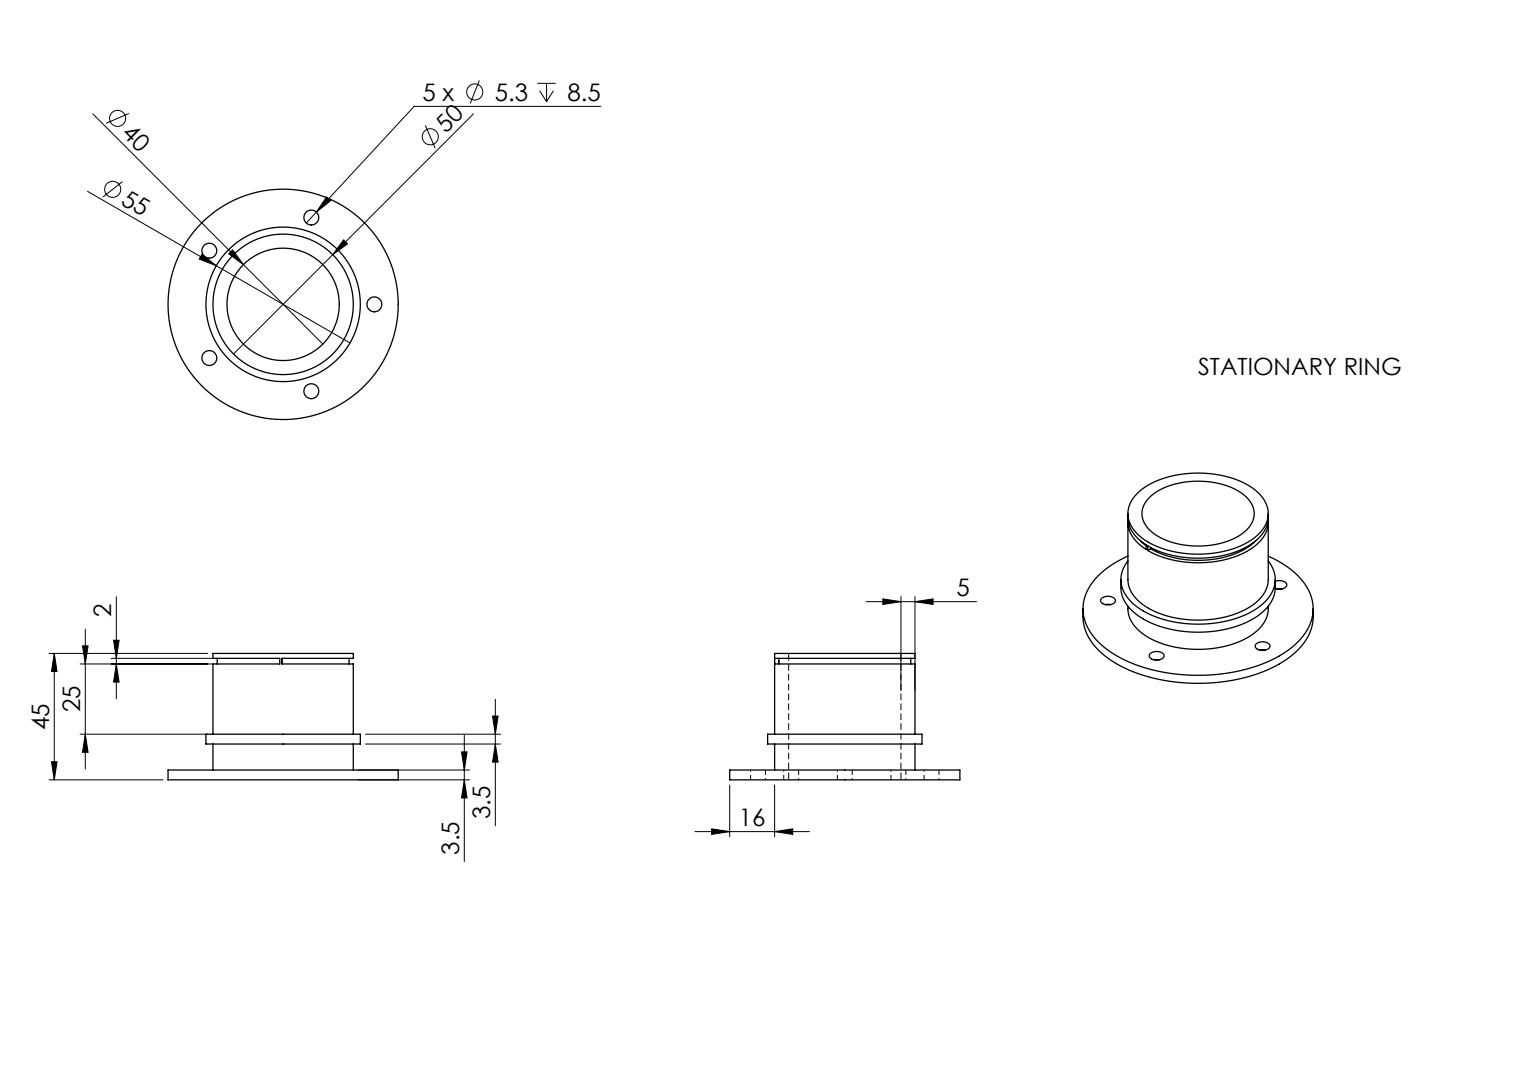
ISO-10303-21;
HEADER;
FILE_DESCRIPTION (('STEP AP214'),
    '1' );
FILE_NAME ('stationary ring.step',
    '2026-10-24T07:08:27',
    ( '' ),
    ( '' ),
    'SwSTEP 2.0',
    'SolidWorks 2026',
    '' );
FILE_SCHEMA (( 'AUTOMOTIVE_DESIGN' ));
ENDSEC;

DATA;
#9=DIRECTION ( 'NONE',  ( 0.000000000000000000, 0.000000000000000000, 1.000000000000000000 ) ) ;
#18=DIRECTION ( 'NONE',  ( 0.000000000000000000, 0.000000000000000000, 1.000000000000000000 ) ) ;
#72=VERTEX_POINT ( 'NONE', #15446 ) ;
#131=ORIENTED_EDGE ( 'NONE', *, *, #5631, .T. ) ;
#137=CARTESIAN_POINT ( 'NONE',  ( -26.29305231718568336, -30.00000000000000000, -19.10302069950552095 ) ) ;
#165=DIRECTION ( 'NONE',  ( 0.000000000000000000, 0.000000000000000000, 1.000000000000000000 ) ) ;
#167=ORIENTED_EDGE ( 'NONE', *, *, #9471, .T. ) ;
#213=CARTESIAN_POINT ( 'NONE',  ( 5.021051876504148963E-15, -26.50000000000000000, 41.00000000000000000 ) ) ;
#243=VERTEX_POINT ( 'NONE', #16663 ) ;
#248=AXIS2_PLACEMENT_3D ( 'NONE', #8151, #16908, #9666 ) ;
#256=EDGE_LOOP ( 'NONE', ( #13526, #15822 ) ) ;
#283=EDGE_CURVE ( 'NONE', #12652, #8705, #12569, .T. ) ;
#288=DIRECTION ( 'NONE',  ( 0.000000000000000000, 0.000000000000000000, 1.000000000000000000 ) ) ;
#294=CIRCLE ( 'NONE', #10631, 2.649999999999999467 ) ;
#295=EDGE_CURVE ( 'NONE', #2351, #16747, #1024, .T. ) ;
#300=CARTESIAN_POINT ( 'NONE',  ( -23.48826165280196321, 13.24999999999999467, -0.7426739052322690604 ) ) ;
#310=EDGE_LOOP ( 'NONE', ( #17511, #1241, #2457, #12125 ) ) ;
#330=ORIENTED_EDGE ( 'NONE', *, *, #18226, .F. ) ;
#331=DIRECTION ( 'NONE',  ( 0.000000000000000000, 0.000000000000000000, 1.000000000000000000 ) ) ;
#333=DIRECTION ( 'NONE',  ( 0.000000000000000000, 1.000000000000000000, 0.000000000000000000 ) ) ;
#368=DIRECTION ( 'NONE',  ( 0.000000000000000000, -0.000000000000000000, -1.000000000000000000 ) ) ;
#403=ORIENTED_EDGE ( 'NONE', *, *, #7543, .T. ) ;
#420=CARTESIAN_POINT ( 'NONE',  ( 32.50000000000000000, -30.00000000000000000, 3.680389326632394941E-13 ) ) ;
#443=DIRECTION ( 'NONE',  ( -0.000000000000000000, 1.000000000000000000, -0.000000000000000000 ) ) ;
#458=DIRECTION ( 'NONE',  ( 0.000000000000000000, 1.000000000000000000, 0.000000000000000000 ) ) ;
#463=CARTESIAN_POINT ( 'NONE',  ( 0.000000000000000000, -30.00000000000000000, 0.000000000000000000 ) ) ;
#468=ORIENTED_EDGE ( 'NONE', *, *, #14255, .T. ) ;
#470=DIRECTION ( 'NONE',  ( 0.000000000000000000, 0.000000000000000000, 1.000000000000000000 ) ) ;
#480=DIRECTION ( 'NONE',  ( 0.000000000000000000, 0.000000000000000000, 1.000000000000000000 ) ) ;
#502=AXIS2_PLACEMENT_3D ( 'NONE', #14003, #960, #12568 ) ;
#505=DIRECTION ( 'NONE',  ( -0.000000000000000000, 1.000000000000000000, -0.000000000000000000 ) ) ;
#522=DIRECTION ( 'NONE',  ( 0.000000000000000000, 0.000000000000000000, 1.000000000000000000 ) ) ;
#528=AXIS2_PLACEMENT_3D ( 'NONE', #15509, #8361, #6654 ) ;
#576=EDGE_LOOP ( 'NONE', ( #11256, #8349, #6691, #4842 ) ) ;
#614=EDGE_LOOP ( 'NONE', ( #7993, #13909, #15314, #4933 ) ) ;
#616=CYLINDRICAL_SURFACE ( 'NONE', #6258, 2.649999999999999467 ) ;
#631=ORIENTED_EDGE ( 'NONE', *, *, #7642, .T. ) ;
#645=VERTEX_POINT ( 'NONE', #15002 ) ;
#647=ADVANCED_FACE ( 'NONE', ( #12940 ), #11765, .T. ) ;
#718=CIRCLE ( 'NONE', #11362, 2.649999999999995914 ) ;
#737=( GEOMETRIC_REPRESENTATION_CONTEXT ( 3 ) GLOBAL_UNCERTAINTY_ASSIGNED_CONTEXT ( ( #6522 ) ) GLOBAL_UNIT_ASSIGNED_CONTEXT ( ( #17644, #7438, #13541 ) ) REPRESENTATION_CONTEXT ( 'NONE', 'WORKASPACE' ) );
#759=ORIENTED_EDGE ( 'NONE', *, *, #6952, .F. ) ;
#769=DIRECTION ( 'NONE',  ( 0.000000000000000000, 0.000000000000000000, 1.000000000000000000 ) ) ;
#786=AXIS2_PLACEMENT_3D ( 'NONE', #10064, #2821, #8624 ) ;
#790=CARTESIAN_POINT ( 'NONE',  ( 32.50000000000000000, -26.50000000000000000, -2.649999999999631317 ) ) ;
#799=DIRECTION ( 'NONE',  ( 1.000000000000000000, 0.000000000000000000, 0.000000000000000000 ) ) ;
#819=CIRCLE ( 'NONE', #9937, 25.00000000000000000 ) ;
#824=EDGE_CURVE ( 'NONE', #3056, #8661, #8769, .T. ) ;
#836=DIRECTION ( 'NONE',  ( 0.9995004958639132076, 0.000000000000000000, 0.03160314490350067673 ) ) ;
#849=DIRECTION ( 'NONE',  ( 0.000000000000000000, 0.000000000000000000, 1.000000000000000000 ) ) ;
#856=FACE_OUTER_BOUND ( 'NONE', #1144, .T. ) ;
#904=DIRECTION ( 'NONE',  ( 0.9995004958639132076, 0.000000000000000000, 0.03160314490350067673 ) ) ;
#911=CARTESIAN_POINT ( 'NONE',  ( 0.000000000000000000, -17.25000000000000355, 0.000000000000000000 ) ) ;
#932=PLANE ( 'NONE',  #17225 ) ;
#960=DIRECTION ( 'NONE',  ( 0.000000000000000000, -1.000000000000000000, 0.000000000000000000 ) ) ;
#995=AXIS2_PLACEMENT_3D ( 'NONE', #17671, #3385, #1944 ) ;
#998=DIRECTION ( 'NONE',  ( 0.000000000000000000, 1.000000000000000000, 0.000000000000000000 ) ) ;
#1008=CARTESIAN_POINT ( 'NONE',  ( 32.50000000000000000, -30.00000000000000000, 3.680389326632394941E-13 ) ) ;
#1009=CIRCLE ( 'NONE', #13174, 2.649999999999999467 ) ;
#1011=CLOSED_SHELL ( 'NONE', ( #7441, #11689, #11568, #2661, #16694, #4242, #6924, #17624, #7600, #3905, #9825, #4801, #9295, #17673, #7168, #6200, #11234, #2883, #16242, #7379, #4112, #1234, #14456, #2013, #11918, #5051, #647, #1767, #1331, #17222, #4597, #7891, #15182 ) ) ;
#1024=CIRCLE ( 'NONE', #4368, 25.00000000000000000 ) ;
#1044=ORIENTED_EDGE ( 'NONE', *, *, #4817, .F. ) ;
#1071=CYLINDRICAL_SURFACE ( 'NONE', #11264, 25.00000000000000000 ) ;
#1090=DIRECTION ( 'NONE',  ( 1.000000000000000000, 0.000000000000000000, 0.000000000000000000 ) ) ;
#1123=DIRECTION ( 'NONE',  ( 0.000000000000000000, 1.000000000000000000, 0.000000000000000000 ) ) ;
#1133=EDGE_LOOP ( 'NONE', ( #14796, #17474, #167, #6880 ) ) ;
#1144=EDGE_LOOP ( 'NONE', ( #12663, #16681, #4780, #9245 ) ) ;
#1149=VECTOR ( 'NONE', #3764, 1000.000000000000000 ) ;
#1163=DIRECTION ( 'NONE',  ( 0.9995004958639132076, 0.000000000000000000, 0.03160314490350067673 ) ) ;
#1178=VERTEX_POINT ( 'NONE', #8655 ) ;
#1208=DIRECTION ( 'NONE',  ( -0.000000000000000000, -1.000000000000000000, 0.000000000000000000 ) ) ;
#1212=CARTESIAN_POINT ( 'NONE',  ( 0.000000000000000000, 15.00000000000000000, 0.000000000000000000 ) ) ;
#1221=ORIENTED_EDGE ( 'NONE', *, *, #283, .T. ) ;
#1233=CIRCLE ( 'NONE', #13693, 2.649999999999999467 ) ;
#1234=ADVANCED_FACE ( 'NONE', ( #6958, #5614 ), #17247, .T. ) ;
#1237=ORIENTED_EDGE ( 'NONE', *, *, #10447, .F. ) ;
#1241=ORIENTED_EDGE ( 'NONE', *, *, #10447, .T. ) ;
#1252=DIRECTION ( 'NONE',  ( -0.000000000000000000, 1.000000000000000000, -0.000000000000000000 ) ) ;
#1253=CARTESIAN_POINT ( 'NONE',  ( 3.061616997868383043E-15, -17.25000000000000355, -25.00000000000000000 ) ) ;
#1268=FACE_OUTER_BOUND ( 'NONE', #15069, .T. ) ;
#1269=CARTESIAN_POINT ( 'NONE',  ( 23.48826165280196321, 13.24999999999999467, 0.7426739052322660628 ) ) ;
#1291=EDGE_CURVE ( 'NONE', #9889, #9794, #9042, .T. ) ;
#1314=ORIENTED_EDGE ( 'NONE', *, *, #6426, .T. ) ;
#1331=ADVANCED_FACE ( 'NONE', ( #10924 ), #16748, .F. ) ;
#1350=COLOUR_RGB ( '',0.8941176470588234615, 0.8941176470588234615, 0.8941176470588234615 ) ;
#1371=VECTOR ( 'NONE', #15439, 1000.000000000000000 ) ;
#1390=CIRCLE ( 'NONE', #4734, 2.649999999999999467 ) ;
#1430=DIRECTION ( 'NONE',  ( 0.000000000000000000, 1.000000000000000000, 0.000000000000000000 ) ) ;
#1433=CARTESIAN_POINT ( 'NONE',  ( 0.000000000000000000, 11.24999999999999645, 0.000000000000000000 ) ) ;
#1466=SHAPE_DEFINITION_REPRESENTATION ( #10584, #16742 ) ;
#1491=VECTOR ( 'NONE', #18744, 1000.000000000000000 ) ;
#1492=CARTESIAN_POINT ( 'NONE',  ( -26.29305231718568336, -30.00000000000000000, -21.75302069950551953 ) ) ;
#1506=ORIENTED_EDGE ( 'NONE', *, *, #17282, .F. ) ;
#1512=ORIENTED_EDGE ( 'NONE', *, *, #4100, .T. ) ;
#1520=CARTESIAN_POINT ( 'NONE',  ( 10.04305231718579705, -26.50000000000000000, 30.90933677959249337 ) ) ;
#1534=VECTOR ( 'NONE', #18328, 1000.000000000000000 ) ;
#1576=EDGE_CURVE ( 'NONE', #16034, #9749, #10261, .T. ) ;
#1646=DIRECTION ( 'NONE',  ( 0.000000000000000000, 1.000000000000000000, 0.000000000000000000 ) ) ;
#1652=FACE_OUTER_BOUND ( 'NONE', #6703, .T. ) ;
#1693=DIRECTION ( 'NONE',  ( 0.000000000000000000, 1.000000000000000000, 0.000000000000000000 ) ) ;
#1729=ORIENTED_EDGE ( 'NONE', *, *, #8148, .T. ) ;
#1735=ORIENTED_EDGE ( 'NONE', *, *, #824, .F. ) ;
#1739=CARTESIAN_POINT ( 'NONE',  ( 10.04305231718605285, -26.50000000000000000, -30.90933677959240811 ) ) ;
#1741=AXIS2_PLACEMENT_3D ( 'NONE', #10000, #3504, #8070 ) ;
#1767=ADVANCED_FACE ( 'NONE', ( #15350 ), #18219, .F. ) ;
#1771=EDGE_CURVE ( 'NONE', #6586, #2692, #8142, .T. ) ;
#1772=CIRCLE ( 'NONE', #8168, 25.00000000000000000 ) ;
#1787=EDGE_CURVE ( 'NONE', #9218, #9749, #16993, .T. ) ;
#1819=FACE_BOUND ( 'NONE', #13502, .T. ) ;
#1822=DIRECTION ( 'NONE',  ( 0.000000000000000000, 0.000000000000000000, 1.000000000000000000 ) ) ;
#1836=LINE ( 'NONE', #14981, #15092 ) ;
#1929=LINE ( 'NONE', #7730, #2930 ) ;
#1944=DIRECTION ( 'NONE',  ( 0.9995004958639130965, 0.000000000000000000, 0.03160314490350068367 ) ) ;
#1955=ORIENTED_EDGE ( 'NONE', *, *, #5164, .T. ) ;
#2013=ADVANCED_FACE ( 'NONE', ( #3443 ), #15158, .T. ) ;
#2032=DIRECTION ( 'NONE',  ( 0.000000000000000000, 0.000000000000000000, 1.000000000000000000 ) ) ;
#2045=DIRECTION ( 'NONE',  ( -0.000000000000000000, 1.000000000000000000, -0.000000000000000000 ) ) ;
#2074=VECTOR ( 'NONE', #10954, 1000.000000000000000 ) ;
#2083=LINE ( 'NONE', #12177, #15046 ) ;
#2131=CARTESIAN_POINT ( 'NONE',  ( 0.000000000000000000, -13.75000000000000355, 27.50000000000000000 ) ) ;
#2161=LINE ( 'NONE', #12448, #9732 ) ;
#2163=CIRCLE ( 'NONE', #10382, 2.649999999999999467 ) ;
#2170=DIRECTION ( 'NONE',  ( 0.000000000000000000, 0.000000000000000000, 1.000000000000000000 ) ) ;
#2173=DIRECTION ( 'NONE',  ( -0.000000000000000000, 1.000000000000000000, -0.000000000000000000 ) ) ;
#2230=CARTESIAN_POINT ( 'NONE',  ( 0.000000000000000000, 15.00000000000000000, 20.00000000000000000 ) ) ;
#2245=CYLINDRICAL_SURFACE ( 'NONE', #9597, 23.50000000000001066 ) ;
#2274=CIRCLE ( 'NONE', #3803, 2.649999999999999467 ) ;
#2277=DIRECTION ( 'NONE',  ( 0.000000000000000000, 0.000000000000000000, 1.000000000000000000 ) ) ;
#2294=VECTOR ( 'NONE', #10245, 1000.000000000000000 ) ;
#2303=DIRECTION ( 'NONE',  ( 0.9995004958639130965, 0.000000000000000000, 0.03160314490350068367 ) ) ;
#2308=CARTESIAN_POINT ( 'NONE',  ( -26.29305231718568336, -30.00000000000000000, -16.45302069950552237 ) ) ;
#2342=ORIENTED_EDGE ( 'NONE', *, *, #6563, .T. ) ;
#2351=VERTEX_POINT ( 'NONE', #1253 ) ;
#2443=CARTESIAN_POINT ( 'NONE',  ( 3.367778697655221307E-15, -13.75000000000000355, -27.50000000000000000 ) ) ;
#2448=DIRECTION ( 'NONE',  ( 0.000000000000000000, 0.000000000000000000, 1.000000000000000000 ) ) ;
#2452=AXIS2_PLACEMENT_3D ( 'NONE', #15849, #11469, #1090 ) ;
#2457=ORIENTED_EDGE ( 'NONE', *, *, #15300, .F. ) ;
#2531=VERTEX_POINT ( 'NONE', #17790 ) ;
#2541=PRODUCT_DEFINITION_CONTEXT ( 'detailed design', #9758, 'design' ) ;
#2549=EDGE_CURVE ( 'NONE', #8661, #3056, #6044, .T. ) ;
#2560=ORIENTED_EDGE ( 'NONE', *, *, #6446, .F. ) ;
#2570=DIRECTION ( 'NONE',  ( -0.000000000000000000, -1.000000000000000000, -0.000000000000000000 ) ) ;
#2582=LINE ( 'NONE', #2690, #16318 ) ;
#2590=EDGE_CURVE ( 'NONE', #5558, #16747, #12648, .T. ) ;
#2595=DIRECTION ( 'NONE',  ( 0.000000000000000000, 0.000000000000000000, 1.000000000000000000 ) ) ;
#2639=ORIENTED_EDGE ( 'NONE', *, *, #16358, .T. ) ;
#2647=ORIENTED_EDGE ( 'NONE', *, *, #6446, .T. ) ;
#2661=ADVANCED_FACE ( 'NONE', ( #856 ), #5123, .F. ) ;
#2677=DIRECTION ( 'NONE',  ( 0.000000000000000000, 0.000000000000000000, 1.000000000000000000 ) ) ;
#2690=CARTESIAN_POINT ( 'NONE',  ( 3.061616997868383043E-15, -30.00000000000000000, -25.00000000000000000 ) ) ;
#2692=VERTEX_POINT ( 'NONE', #11116 ) ;
#2695=DIRECTION ( 'NONE',  ( -0.000000000000000000, 1.000000000000000000, 0.000000000000000000 ) ) ;
#2715=CIRCLE ( 'NONE', #6973, 2.649999999999995914 ) ;
#2720=ORIENTED_EDGE ( 'NONE', *, *, #14352, .F. ) ;
#2723=FACE_OUTER_BOUND ( 'NONE', #12700, .T. ) ;
#2737=DIRECTION ( 'NONE',  ( 0.000000000000000000, 0.000000000000000000, 1.000000000000000000 ) ) ;
#2754=DIRECTION ( 'NONE',  ( 0.000000000000000000, 1.000000000000000000, 0.000000000000000000 ) ) ;
#2764=LINE ( 'NONE', #12948, #2941 ) ;
#2821=DIRECTION ( 'NONE',  ( 0.000000000000000000, -1.000000000000000000, 0.000000000000000000 ) ) ;
#2874=ORIENTED_EDGE ( 'NONE', *, *, #16364, .F. ) ;
#2881=CARTESIAN_POINT ( 'NONE',  ( -26.29305231718568336, -30.00000000000000000, -19.10302069950552095 ) ) ;
#2883=ADVANCED_FACE ( 'NONE', ( #10436 ), #4542, .F. ) ;
#2895=CARTESIAN_POINT ( 'NONE',  ( 2.449293598294706513E-15, 15.00000000000000000, -20.00000000000000000 ) ) ;
#2930=VECTOR ( 'NONE', #505, 1000.000000000000000 ) ;
#2941=VECTOR ( 'NONE', #5714, 1000.000000000000000 ) ;
#3022=CARTESIAN_POINT ( 'NONE',  ( 0.000000000000000000, -13.75000000000000355, 0.000000000000000000 ) ) ;
#3056=VERTEX_POINT ( 'NONE', #13688 ) ;
#3059=CIRCLE ( 'NONE', #10349, 23.50000000000001066 ) ;
#3079=PRESENTATION_STYLE_ASSIGNMENT (( #16125 ) ) ;
#3080=CYLINDRICAL_SURFACE ( 'NONE', #6330, 2.649999999999999467 ) ;
#3083=EDGE_LOOP ( 'NONE', ( #1221, #16532, #13684, #14432, #1506, #13517, #11608, #1237 ) ) ;
#3126=AXIS2_PLACEMENT_3D ( 'NONE', #3946, #13938, #18506 ) ;
#3138=CIRCLE ( 'NONE', #12566, 23.50000000000001066 ) ;
#3162=FILL_AREA_STYLE_COLOUR ( '', #1350 ) ;
#3185=CARTESIAN_POINT ( 'NONE',  ( 0.000000000000000000, -17.25000000000000355, 0.000000000000000000 ) ) ;
#3202=ORIENTED_EDGE ( 'NONE', *, *, #17282, .T. ) ;
#3216=AXIS2_PLACEMENT_3D ( 'NONE', #15972, #12849, #5703 ) ;
#3248=ORIENTED_EDGE ( 'NONE', *, *, #4834, .T. ) ;
#3264=EDGE_CURVE ( 'NONE', #15594, #13366, #11740, .T. ) ;
#3290=ORIENTED_EDGE ( 'NONE', *, *, #16108, .F. ) ;
#3302=EDGE_LOOP ( 'NONE', ( #13752, #17572 ) ) ;
#3347=AXIS2_PLACEMENT_3D ( 'NONE', #5723, #2570, #15537 ) ;
#3363=ORIENTED_EDGE ( 'NONE', *, *, #4070, .F. ) ;
#3385=DIRECTION ( 'NONE',  ( -0.000000000000000000, 1.000000000000000000, 0.000000000000000000 ) ) ;
#3416=DIRECTION ( 'NONE',  ( -0.01515971714484241201, 0.000000000000000000, 0.9998850848853023665 ) ) ;
#3422=FACE_BOUND ( 'NONE', #14128, .T. ) ;
#3429=EDGE_CURVE ( 'NONE', #243, #18412, #12129, .T. ) ;
#3443=FACE_OUTER_BOUND ( 'NONE', #17179, .T. ) ;
#3444=CYLINDRICAL_SURFACE ( 'NONE', #7956, 2.649999999999995914 ) ;
#3449=( NAMED_UNIT ( * ) SI_UNIT ( $, .STERADIAN. ) SOLID_ANGLE_UNIT ( ) );
#3458=( NAMED_UNIT ( * ) SI_UNIT ( $, .STERADIAN. ) SOLID_ANGLE_UNIT ( ) );
#3484=ORIENTED_EDGE ( 'NONE', *, *, #16364, .T. ) ;
#3495=LINE ( 'NONE', #16451, #10796 ) ;
#3503=ORIENTED_EDGE ( 'NONE', *, *, #14588, .T. ) ;
#3504=DIRECTION ( 'NONE',  ( 0.000000000000000000, 1.000000000000000000, 0.000000000000000000 ) ) ;
#3543=AXIS2_PLACEMENT_3D ( 'NONE', #1433, #7237, #18 ) ;
#3561=DIRECTION ( 'NONE',  ( 0.000000000000000000, 0.000000000000000000, 1.000000000000000000 ) ) ;
#3571=CYLINDRICAL_SURFACE ( 'NONE', #5725, 27.50000000000000000 ) ;
#3581=AXIS2_PLACEMENT_3D ( 'NONE', #10797, #9186, #14816 ) ;
#3601=EDGE_CURVE ( 'NONE', #16476, #6965, #11748, .T. ) ;
#3613=VERTEX_POINT ( 'NONE', #16660 ) ;
#3615=DIRECTION ( 'NONE',  ( 0.000000000000000000, 1.000000000000000000, 0.000000000000000000 ) ) ;
#3635=CARTESIAN_POINT ( 'NONE',  ( -26.29305231718584324, -26.50000000000000000, 19.10302069950530779 ) ) ;
#3642=CIRCLE ( 'NONE', #3347, 25.00000000000000000 ) ;
#3660=DIRECTION ( 'NONE',  ( 0.000000000000000000, 1.000000000000000000, 0.000000000000000000 ) ) ;
#3680=UNCERTAINTY_MEASURE_WITH_UNIT (LENGTH_MEASURE( 1.000000000000000082E-05 ), #8870, 'distance_accuracy_value', 'NONE');
#3699=CARTESIAN_POINT ( 'NONE',  ( 32.50000000000000000, -26.50000000000000000, 3.680389326632394941E-13 ) ) ;
#3717=ORIENTED_EDGE ( 'NONE', *, *, #8148, .F. ) ;
#3721=FACE_OUTER_BOUND ( 'NONE', #18727, .T. ) ;
#3764=DIRECTION ( 'NONE',  ( 0.000000000000000000, 1.000000000000000000, 0.000000000000000000 ) ) ;
#3770=ORIENTED_EDGE ( 'NONE', *, *, #2590, .T. ) ;
#3803=AXIS2_PLACEMENT_3D ( 'NONE', #10925, #16749, #2170 ) ;
#3823=AXIS2_PLACEMENT_3D ( 'NONE', #14060, #6530, #11095 ) ;
#3829=DIRECTION ( 'NONE',  ( -0.000000000000000000, -1.000000000000000000, -0.000000000000000000 ) ) ;
#3845=ORIENTED_EDGE ( 'NONE', *, *, #16410, .T. ) ;
#3883=EDGE_CURVE ( 'NONE', #16268, #4068, #5652, .T. ) ;
#3905=ADVANCED_FACE ( 'NONE', ( #17332 ), #13129, .F. ) ;
#3935=CIRCLE ( 'NONE', #13976, 2.649999999999999467 ) ;
#3939=ORIENTED_EDGE ( 'NONE', *, *, #7905, .F. ) ;
#3944=CARTESIAN_POINT ( 'NONE',  ( 32.50000000000000000, -26.50000000000000000, -2.649999999999631317 ) ) ;
#3946=CARTESIAN_POINT ( 'NONE',  ( 0.000000000000000000, -30.00000000000000000, 0.000000000000000000 ) ) ;
#3975=FACE_BOUND ( 'NONE', #256, .T. ) ;
#3998=DIRECTION ( 'NONE',  ( 0.000000000000000000, 0.000000000000000000, 1.000000000000000000 ) ) ;
#4028=EDGE_CURVE ( 'NONE', #13569, #12768, #3495, .T. ) ;
#4044=DIRECTION ( 'NONE',  ( 0.000000000000000000, 0.000000000000000000, 1.000000000000000000 ) ) ;
#4051=ORIENTED_EDGE ( 'NONE', *, *, #18226, .T. ) ;
#4068=VERTEX_POINT ( 'NONE', #6157 ) ;
#4070=EDGE_CURVE ( 'NONE', #4975, #6521, #9290, .T. ) ;
#4100=EDGE_CURVE ( 'NONE', #6721, #12768, #1390, .T. ) ;
#4110=CIRCLE ( 'NONE', #14131, 20.00000000000000000 ) ;
#4112=ADVANCED_FACE ( 'NONE', ( #3975, #9574 ), #932, .F. ) ;
#4125=CARTESIAN_POINT ( 'NONE',  ( 0.000000000000000000, 13.24999999999999467, 0.000000000000000000 ) ) ;
#4131=EDGE_CURVE ( 'NONE', #8705, #8908, #11437, .T. ) ;
#4157=CARTESIAN_POINT ( 'NONE',  ( 0.000000000000000000, -17.25000000000000355, 0.000000000000000000 ) ) ;
#4172=CIRCLE ( 'NONE', #502, 41.00000000000000000 ) ;
#4183=ORIENTED_EDGE ( 'NONE', *, *, #824, .T. ) ;
#4199=DIRECTION ( 'NONE',  ( 0.000000000000000000, 1.000000000000000000, 0.000000000000000000 ) ) ;
#4213=ORIENTED_EDGE ( 'NONE', *, *, #18657, .T. ) ;
#4230=VERTEX_POINT ( 'NONE', #2443 ) ;
#4233=ORIENTED_EDGE ( 'NONE', *, *, #6890, .F. ) ;
#4242=ADVANCED_FACE ( 'NONE', ( #18153 ), #2245, .T. ) ;
#4243=ORIENTED_EDGE ( 'NONE', *, *, #10832, .F. ) ;
#4280=DIRECTION ( 'NONE',  ( 0.000000000000000000, 0.000000000000000000, 1.000000000000000000 ) ) ;
#4308=DIRECTION ( 'NONE',  ( 0.000000000000000000, 0.000000000000000000, -1.000000000000000000 ) ) ;
#4361=DIRECTION ( 'NONE',  ( 0.000000000000000000, 0.000000000000000000, 1.000000000000000000 ) ) ;
#4365=EDGE_CURVE ( 'NONE', #12674, #9439, #5030, .T. ) ;
#4368=AXIS2_PLACEMENT_3D ( 'NONE', #4755, #6278, #10837 ) ;
#4380=DIRECTION ( 'NONE',  ( 0.000000000000000000, -1.000000000000000000, 0.000000000000000000 ) ) ;
#4402=DIRECTION ( 'NONE',  ( 0.000000000000000000, 0.000000000000000000, 1.000000000000000000 ) ) ;
#4404=EDGE_LOOP ( 'NONE', ( #5392, #18272 ) ) ;
#4440=ORIENTED_EDGE ( 'NONE', *, *, #15992, .T. ) ;
#4457=CARTESIAN_POINT ( 'NONE',  ( 0.000000000000000000, 13.24999999999999467, 0.000000000000000000 ) ) ;
#4493=CARTESIAN_POINT ( 'NONE',  ( 0.000000000000000000, -30.00000000000000000, 0.000000000000000000 ) ) ;
#4501=LINE ( 'NONE', #213, #17922 ) ;
#4517=AXIS2_PLACEMENT_3D ( 'NONE', #2881, #10122, #2595 ) ;
#4523=DIRECTION ( 'NONE',  ( 0.000000000000000000, -1.000000000000000000, 0.000000000000000000 ) ) ;
#4542=CYLINDRICAL_SURFACE ( 'NONE', #14192, 20.00000000000000000 ) ;
#4585=FACE_OUTER_BOUND ( 'NONE', #12863, .T. ) ;
#4591=EDGE_CURVE ( 'NONE', #6386, #6721, #12602, .T. ) ;
#4592=DIRECTION ( 'NONE',  ( 0.000000000000000000, 1.000000000000000000, 0.000000000000000000 ) ) ;
#4597=ADVANCED_FACE ( 'NONE', ( #7848 ), #616, .F. ) ;
#4618=ORIENTED_EDGE ( 'NONE', *, *, #13445, .T. ) ;
#4627=ORIENTED_EDGE ( 'NONE', *, *, #2549, .T. ) ;
#4634=ORIENTED_EDGE ( 'NONE', *, *, #6742, .T. ) ;
#4724=CARTESIAN_POINT ( 'NONE',  ( -26.29305231718568336, -26.50000000000000000, -19.10302069950552095 ) ) ;
#4734=AXIS2_PLACEMENT_3D ( 'NONE', #4724, #443, #6356 ) ;
#4755=CARTESIAN_POINT ( 'NONE',  ( 0.000000000000000000, -17.25000000000000355, 0.000000000000000000 ) ) ;
#4775=SURFACE_STYLE_FILL_AREA ( #16406 ) ;
#4776=CARTESIAN_POINT ( 'NONE',  ( 0.000000000000000000, -30.00000000000000000, 25.00000000000000000 ) ) ;
#4780=ORIENTED_EDGE ( 'NONE', *, *, #8755, .T. ) ;
#4785=( LENGTH_UNIT ( ) NAMED_UNIT ( * ) SI_UNIT ( .MILLI., .METRE. ) );
#4793=ORIENTED_EDGE ( 'NONE', *, *, #12813, .F. ) ;
#4797=CARTESIAN_POINT ( 'NONE',  ( 10.04305231718579705, -26.50000000000000000, 30.90933677959249337 ) ) ;
#4801=ADVANCED_FACE ( 'NONE', ( #3721 ), #9518, .T. ) ;
#4817=EDGE_CURVE ( 'NONE', #12768, #6721, #15427, .T. ) ;
#4834=EDGE_CURVE ( 'NONE', #13484, #12910, #4172, .T. ) ;
#4836=DIRECTION ( 'NONE',  ( 0.000000000000000000, 1.000000000000000000, 0.000000000000000000 ) ) ;
#4842=ORIENTED_EDGE ( 'NONE', *, *, #5631, .F. ) ;
#4844=CARTESIAN_POINT ( 'NONE',  ( -26.29305231718584324, -30.00000000000000000, 16.45302069950530566 ) ) ;
#4871=SURFACE_SIDE_STYLE ('',( #4775 ) ) ;
#4893=EDGE_LOOP ( 'NONE', ( #6155, #8486 ) ) ;
#4905=FACE_OUTER_BOUND ( 'NONE', #18171, .T. ) ;
#4918=ORIENTED_EDGE ( 'NONE', *, *, #16108, .T. ) ;
#4933=ORIENTED_EDGE ( 'NONE', *, *, #1576, .T. ) ;
#4957=EDGE_CURVE ( 'NONE', #243, #12652, #2764, .T. ) ;
#4975=VERTEX_POINT ( 'NONE', #10090 ) ;
#5030=CIRCLE ( 'NONE', #16006, 25.00000000000000000 ) ;
#5051=ADVANCED_FACE ( 'NONE', ( #10551 ), #6078, .F. ) ;
#5069=DIRECTION ( 'NONE',  ( -0.000000000000000000, -1.000000000000000000, 0.000000000000000000 ) ) ;
#5077=DIRECTION ( 'NONE',  ( 0.9995004958639132076, 0.000000000000000000, 0.03160314490350067673 ) ) ;
#5123=CYLINDRICAL_SURFACE ( 'NONE', #17011, 2.649999999999995914 ) ;
#5130=ORIENTED_EDGE ( 'NONE', *, *, #4365, .T. ) ;
#5139=DIRECTION ( 'NONE',  ( -0.000000000000000000, 1.000000000000000000, -0.000000000000000000 ) ) ;
#5164=EDGE_CURVE ( 'NONE', #6521, #1178, #17268, .T. ) ;
#5178=ORIENTED_EDGE ( 'NONE', *, *, #4028, .T. ) ;
#5211=CARTESIAN_POINT ( 'NONE',  ( 0.000000000000000000, 15.00000000000000000, 0.000000000000000000 ) ) ;
#5275=AXIS2_PLACEMENT_3D ( 'NONE', #10333, #4523, #7460 ) ;
#5303=LINE ( 'NONE', #11111, #16882 ) ;
#5314=CARTESIAN_POINT ( 'NONE',  ( 10.04305231718605285, -26.50000000000000000, -30.90933677959240811 ) ) ;
#5348=DIRECTION ( 'NONE',  ( 0.000000000000000000, 0.000000000000000000, 1.000000000000000000 ) ) ;
#5356=ADVANCED_BREP_SHAPE_REPRESENTATION ( '', ( #9701, #8017 ), #737 ) ;
#5376=CARTESIAN_POINT ( 'NONE',  ( -26.29305231718584324, -26.50000000000000000, 21.75302069950530637 ) ) ;
#5392=ORIENTED_EDGE ( 'NONE', *, *, #13718, .T. ) ;
#5411=DIRECTION ( 'NONE',  ( 0.9995004958639132076, 0.000000000000000000, 0.03160314490350067673 ) ) ;
#5415=EDGE_LOOP ( 'NONE', ( #13884, #8621, #11743, #1512 ) ) ;
#5428=CARTESIAN_POINT ( 'NONE',  ( 0.000000000000000000, 11.24999999999999645, 0.000000000000000000 ) ) ;
#5435=VERTEX_POINT ( 'NONE', #16374 ) ;
#5447=ORIENTED_EDGE ( 'NONE', *, *, #4957, .F. ) ;
#5456=CIRCLE ( 'NONE', #16092, 25.00000000000000000 ) ;
#5465=CARTESIAN_POINT ( 'NONE',  ( 10.04305231718605285, -30.00000000000000000, -30.90933677959240811 ) ) ;
#5474=DIRECTION ( 'NONE',  ( 0.000000000000000000, 1.000000000000000000, 0.000000000000000000 ) ) ;
#5482=AXIS2_PLACEMENT_3D ( 'NONE', #6517, #15104, #16618 ) ;
#5540=CARTESIAN_POINT ( 'NONE',  ( 0.000000000000000000, 11.24999999999999467, 0.000000000000000000 ) ) ;
#5558=VERTEX_POINT ( 'NONE', #8176 ) ;
#5581=ORIENTED_EDGE ( 'NONE', *, *, #2590, .F. ) ;
#5596=DIRECTION ( 'NONE',  ( 0.000000000000000000, 1.000000000000000000, 0.000000000000000000 ) ) ;
#5614=FACE_OUTER_BOUND ( 'NONE', #8466, .T. ) ;
#5631=EDGE_CURVE ( 'NONE', #17331, #9794, #7105, .T. ) ;
#5632=ORIENTED_EDGE ( 'NONE', *, *, #18805, .T. ) ;
#5637=CIRCLE ( 'NONE', #16281, 2.649999999999995914 ) ;
#5652=CIRCLE ( 'NONE', #3216, 2.649999999999999467 ) ;
#5703=DIRECTION ( 'NONE',  ( 0.000000000000000000, 0.000000000000000000, 1.000000000000000000 ) ) ;
#5714=DIRECTION ( 'NONE',  ( 0.000000000000000000, 1.000000000000000000, 0.000000000000000000 ) ) ;
#5723=CARTESIAN_POINT ( 'NONE',  ( 0.000000000000000000, 11.24999999999999645, 0.000000000000000000 ) ) ;
#5725=AXIS2_PLACEMENT_3D ( 'NONE', #911, #15469, #11065 ) ;
#5756=EDGE_LOOP ( 'NONE', ( #3363, #759, #1729, #4634 ) ) ;
#5810=CARTESIAN_POINT ( 'NONE',  ( 0.000000000000000000, -26.50000000000000000, 0.000000000000000000 ) ) ;
#5830=DIRECTION ( 'NONE',  ( 0.000000000000000000, 0.000000000000000000, 1.000000000000000000 ) ) ;
#5834=DIRECTION ( 'NONE',  ( -0.000000000000000000, -1.000000000000000000, -0.000000000000000000 ) ) ;
#5914=DIRECTION ( 'NONE',  ( 0.000000000000000000, 1.000000000000000000, 0.000000000000000000 ) ) ;
#5926=DIRECTION ( 'NONE',  ( 0.000000000000000000, 1.000000000000000000, 0.000000000000000000 ) ) ;
#5970=CIRCLE ( 'NONE', #8416, 41.00000000000000000 ) ;
#5975=ORIENTED_EDGE ( 'NONE', *, *, #12831, .F. ) ;
#5982=FACE_OUTER_BOUND ( 'NONE', #17091, .T. ) ;
#5985=CYLINDRICAL_SURFACE ( 'NONE', #13306, 2.649999999999999467 ) ;
#5992=EDGE_CURVE ( 'NONE', #17369, #72, #16669, .T. ) ;
#5996=AXIS2_PLACEMENT_3D ( 'NONE', #1520, #15553, #9 ) ;
#6044=CIRCLE ( 'NONE', #13043, 20.00000000000000000 ) ;
#6061=CARTESIAN_POINT ( 'NONE',  ( 0.000000000000000000, -30.00000000000000000, 0.000000000000000000 ) ) ;
#6066=CARTESIAN_POINT ( 'NONE',  ( 10.04305231718579705, -26.50000000000000000, 28.25933677959249835 ) ) ;
#6069=ORIENTED_EDGE ( 'NONE', *, *, #8644, .F. ) ;
#6077=EDGE_LOOP ( 'NONE', ( #10014, #4213 ) ) ;
#6078=PLANE ( 'NONE',  #16629 ) ;
#6109=EDGE_LOOP ( 'NONE', ( #12115, #2874 ) ) ;
#6126=CYLINDRICAL_SURFACE ( 'NONE', #14673, 2.649999999999999467 ) ;
#6152=DIRECTION ( 'NONE',  ( 0.000000000000000000, 1.000000000000000000, 0.000000000000000000 ) ) ;
#6155=ORIENTED_EDGE ( 'NONE', *, *, #14448, .F. ) ;
#6157=CARTESIAN_POINT ( 'NONE',  ( -26.29305231718584324, -30.00000000000000000, 21.75302069950530637 ) ) ;
#6162=AXIS2_PLACEMENT_3D ( 'NONE', #9836, #5069, #904 ) ;
#6179=CARTESIAN_POINT ( 'NONE',  ( -26.29305231718584324, -26.50000000000000000, 19.10302069950530779 ) ) ;
#6183=CARTESIAN_POINT ( 'NONE',  ( 0.000000000000000000, 13.24999999999999822, 0.000000000000000000 ) ) ;
#6200=ADVANCED_FACE ( 'NONE', ( #13563 ), #16423, .T. ) ;
#6201=SHAPE_REPRESENTATION_RELATIONSHIP ( 'NONE' , 'NONE' ,  #16742, #5356 ) ;
#6223=DIRECTION ( 'NONE',  ( 0.000000000000000000, 0.000000000000000000, 1.000000000000000000 ) ) ;
#6258=AXIS2_PLACEMENT_3D ( 'NONE', #6421, #7938, #8029 ) ;
#6264=AXIS2_PLACEMENT_3D ( 'NONE', #10502, #8804, #331 ) ;
#6278=DIRECTION ( 'NONE',  ( -0.000000000000000000, -1.000000000000000000, -0.000000000000000000 ) ) ;
#6298=ORIENTED_EDGE ( 'NONE', *, *, #18060, .T. ) ;
#6307=AXIS2_PLACEMENT_3D ( 'NONE', #4797, #12028, #6223 ) ;
#6309=DIRECTION ( 'NONE',  ( -0.000000000000000000, -1.000000000000000000, -0.000000000000000000 ) ) ;
#6330=AXIS2_PLACEMENT_3D ( 'NONE', #17816, #14883, #10315 ) ;
#6356=DIRECTION ( 'NONE',  ( 0.000000000000000000, 0.000000000000000000, 1.000000000000000000 ) ) ;
#6386=VERTEX_POINT ( 'NONE', #2308 ) ;
#6391=CARTESIAN_POINT ( 'NONE',  ( -1.200950573245989306, 13.24999999999999822, 24.97113769375797432 ) ) ;
#6395=MECHANICAL_DESIGN_GEOMETRIC_PRESENTATION_REPRESENTATION('',(#16446),#8532);
#6421=CARTESIAN_POINT ( 'NONE',  ( -26.29305231718568336, -26.50000000000000000, -19.10302069950552095 ) ) ;
#6426=EDGE_CURVE ( 'NONE', #9272, #10759, #7860, .T. ) ;
#6446=EDGE_CURVE ( 'NONE', #13569, #6386, #9077, .T. ) ;
#6451=AXIS2_PLACEMENT_3D ( 'NONE', #5810, #4380, #17518 ) ;
#6476=ORIENTED_EDGE ( 'NONE', *, *, #8643, .F. ) ;
#6479=DIRECTION ( 'NONE',  ( 0.000000000000000000, 1.000000000000000000, 0.000000000000000000 ) ) ;
#6504=CARTESIAN_POINT ( 'NONE',  ( 0.000000000000000000, 15.00000000000000000, 0.000000000000000000 ) ) ;
#6505=ORIENTED_EDGE ( 'NONE', *, *, #15300, .T. ) ;
#6517=CARTESIAN_POINT ( 'NONE',  ( 0.000000000000000000, -30.00000000000000000, 0.000000000000000000 ) ) ;
#6521=VERTEX_POINT ( 'NONE', #7261 ) ;
#6522=UNCERTAINTY_MEASURE_WITH_UNIT (LENGTH_MEASURE( 1.000000000000000082E-05 ), #17644, 'distance_accuracy_value', 'NONE');
#6527=CARTESIAN_POINT ( 'NONE',  ( 10.04305231718579705, -30.00000000000000000, 33.55933677959249195 ) ) ;
#6530=DIRECTION ( 'NONE',  ( -0.000000000000000000, -1.000000000000000000, -0.000000000000000000 ) ) ;
#6538=VECTOR ( 'NONE', #7577, 1000.000000000000000 ) ;
#6541=ORIENTED_EDGE ( 'NONE', *, *, #14187, .T. ) ;
#6563=EDGE_CURVE ( 'NONE', #17369, #12910, #4501, .T. ) ;
#6586=VERTEX_POINT ( 'NONE', #17814 ) ;
#6589=ORIENTED_EDGE ( 'NONE', *, *, #13220, .F. ) ;
#6591=CARTESIAN_POINT ( 'NONE',  ( 0.000000000000000000, -26.50000000000000000, 0.000000000000000000 ) ) ;
#6609=CARTESIAN_POINT ( 'NONE',  ( 0.000000000000000000, 13.24999999999999467, 0.000000000000000000 ) ) ;
#6615=EDGE_LOOP ( 'NONE', ( #1735, #4440, #3484, #10637 ) ) ;
#6627=EDGE_LOOP ( 'NONE', ( #10421, #15175, #11949, #7657, #9600, #2720, #6541, #7935, #4793, #10819, #5447, #13324 ) ) ;
#6651=DIRECTION ( 'NONE',  ( 1.000000000000000000, 0.000000000000000000, 0.000000000000000000 ) ) ;
#6654=DIRECTION ( 'NONE',  ( 0.04803802292983955918, 0.000000000000000000, -0.9988455077503187729 ) ) ;
#6691=ORIENTED_EDGE ( 'NONE', *, *, #1291, .T. ) ;
#6700=DIRECTION ( 'NONE',  ( 0.000000000000000000, 0.000000000000000000, 1.000000000000000000 ) ) ;
#6703=EDGE_LOOP ( 'NONE', ( #13405, #7419, #1955, #3717 ) ) ;
#6717=LINE ( 'NONE', #14047, #7177 ) ;
#6721=VERTEX_POINT ( 'NONE', #15060 ) ;
#6728=ORIENTED_EDGE ( 'NONE', *, *, #9575, .F. ) ;
#6742=EDGE_CURVE ( 'NONE', #1178, #6521, #2715, .T. ) ;
#6776=AXIS2_PLACEMENT_3D ( 'NONE', #137, #1646, #18452 ) ;
#6807=CARTESIAN_POINT ( 'NONE',  ( -1.128893538851230005, 11.24999999999999467, 23.47286943213250154 ) ) ;
#6808=DIRECTION ( 'NONE',  ( 0.000000000000000000, 1.000000000000000000, 0.000000000000000000 ) ) ;
#6813=CARTESIAN_POINT ( 'NONE',  ( 0.000000000000000000, 11.24999999999999467, 0.000000000000000000 ) ) ;
#6852=DIRECTION ( 'NONE',  ( 0.000000000000000000, 0.000000000000000000, 1.000000000000000000 ) ) ;
#6880=ORIENTED_EDGE ( 'NONE', *, *, #6989, .T. ) ;
#6890=EDGE_CURVE ( 'NONE', #6965, #8582, #3642, .T. ) ;
#6903=DIRECTION ( 'NONE',  ( 0.000000000000000000, 0.000000000000000000, 1.000000000000000000 ) ) ;
#6924=ADVANCED_FACE ( 'NONE', ( #8390 ), #17157, .T. ) ;
#6929=AXIS2_PLACEMENT_3D ( 'NONE', #420, #998, #15193 ) ;
#6942=EDGE_LOOP ( 'NONE', ( #2639, #17115 ) ) ;
#6952=EDGE_CURVE ( 'NONE', #18105, #4975, #10324, .T. ) ;
#6958=FACE_BOUND ( 'NONE', #7211, .T. ) ;
#6963=VECTOR ( 'NONE', #6479, 1000.000000000000000 ) ;
#6965=VERTEX_POINT ( 'NONE', #8488 ) ;
#6973=AXIS2_PLACEMENT_3D ( 'NONE', #16578, #13729, #16867 ) ;
#6978=DIRECTION ( 'NONE',  ( 0.000000000000000000, 1.000000000000000000, 0.000000000000000000 ) ) ;
#6989=EDGE_CURVE ( 'NONE', #12311, #8822, #294, .T. ) ;
#7007=DIRECTION ( 'NONE',  ( 0.9995004958639132076, 0.000000000000000000, 0.03160314490350067673 ) ) ;
#7070=EDGE_LOOP ( 'NONE', ( #13061, #13508, #14373, #13028 ) ) ;
#7105=LINE ( 'NONE', #14436, #16049 ) ;
#7122=CARTESIAN_POINT ( 'NONE',  ( 5.021051876504148963E-15, -26.50000000000000000, 41.00000000000000000 ) ) ;
#7142=AXIS2_PLACEMENT_3D ( 'NONE', #17785, #1693, #13140 ) ;
#7166=EDGE_LOOP ( 'NONE', ( #6728, #8929 ) ) ;
#7168=ADVANCED_FACE ( 'NONE', ( #18429 ), #18340, .T. ) ;
#7177=VECTOR ( 'NONE', #8336, 1000.000000000000000 ) ;
#7187=APPLICATION_CONTEXT ( 'automotive_design' ) ;
#7211=EDGE_LOOP ( 'NONE', ( #5632, #16300 ) ) ;
#7237=DIRECTION ( 'NONE',  ( -0.000000000000000000, -1.000000000000000000, -0.000000000000000000 ) ) ;
#7261=CARTESIAN_POINT ( 'NONE',  ( 10.04305231718579705, -26.50000000000000000, 28.25933677959249835 ) ) ;
#7321=FACE_BOUND ( 'NONE', #6109, .T. ) ;
#7337=DIRECTION ( 'NONE',  ( 0.000000000000000000, 0.000000000000000000, 1.000000000000000000 ) ) ;
#7341=FACE_BOUND ( 'NONE', #6942, .T. ) ;
#7379=ADVANCED_FACE ( 'NONE', ( #2723 ), #17472, .T. ) ;
#7383=LINE ( 'NONE', #14628, #6538 ) ;
#7389=CARTESIAN_POINT ( 'NONE',  ( 3.061616997868383043E-15, -13.75000000000000533, -25.00000000000000000 ) ) ;
#7397=EDGE_LOOP ( 'NONE', ( #2560, #5178, #11606, #17546 ) ) ;
#7408=DIRECTION ( 'NONE',  ( -0.01515971714484241721, 0.000000000000000000, 0.9998850848853023665 ) ) ;
#7419=ORIENTED_EDGE ( 'NONE', *, *, #4070, .T. ) ;
#7438=( NAMED_UNIT ( * ) PLANE_ANGLE_UNIT ( ) SI_UNIT ( $, .RADIAN. ) );
#7441=ADVANCED_FACE ( 'NONE', ( #1652 ), #7461, .F. ) ;
#7460=DIRECTION ( 'NONE',  ( 0.000000000000000000, 0.000000000000000000, -1.000000000000000000 ) ) ;
#7461=CYLINDRICAL_SURFACE ( 'NONE', #6307, 2.649999999999995914 ) ;
#7466=DIRECTION ( 'NONE',  ( 0.000000000000000000, 1.000000000000000000, 0.000000000000000000 ) ) ;
#7513=CYLINDRICAL_SURFACE ( 'NONE', #6451, 41.00000000000000000 ) ;
#7543=EDGE_CURVE ( 'NONE', #13366, #15594, #10868, .T. ) ;
#7563=EDGE_CURVE ( 'NONE', #9218, #14866, #7826, .T. ) ;
#7577=DIRECTION ( 'NONE',  ( 0.000000000000000000, -1.000000000000000000, 0.000000000000000000 ) ) ;
#7600=ADVANCED_FACE ( 'NONE', ( #12310 ), #3571, .T. ) ;
#7603=CARTESIAN_POINT ( 'NONE',  ( -0.3562533529037968383, 11.24999999999999467, 23.49729949480461499 ) ) ;
#7610=FACE_BOUND ( 'NONE', #8033, .T. ) ;
#7617=DIRECTION ( 'NONE',  ( -0.000000000000000000, -1.000000000000000000, -0.000000000000000000 ) ) ;
#7642=EDGE_CURVE ( 'NONE', #645, #9889, #8455, .T. ) ;
#7643=DIRECTION ( 'NONE',  ( 0.9995004958639132076, 0.000000000000000000, 0.03160314490350067673 ) ) ;
#7648=VERTEX_POINT ( 'NONE', #2131 ) ;
#7657=ORIENTED_EDGE ( 'NONE', *, *, #6890, .T. ) ;
#7662=CYLINDRICAL_SURFACE ( 'NONE', #3581, 2.649999999999995914 ) ;
#7689=CARTESIAN_POINT ( 'NONE',  ( 0.000000000000000000, -30.00000000000000000, 0.000000000000000000 ) ) ;
#7717=AXIS2_PLACEMENT_3D ( 'NONE', #17283, #5834, #4402 ) ;
#7730=CARTESIAN_POINT ( 'NONE',  ( 32.50000000000000000, -26.50000000000000000, 2.650000000000367617 ) ) ;
#7767=EDGE_LOOP ( 'NONE', ( #13784, #4051, #12410, #12605, #9262, #4233, #9103, #6476 ) ) ;
#7778=CARTESIAN_POINT ( 'NONE',  ( -0.3562533529037968383, 11.24999999999999467, 23.49729949480461499 ) ) ;
#7802=AXIS2_PLACEMENT_3D ( 'NONE', #13699, #8772, #7337 ) ;
#7809=CARTESIAN_POINT ( 'NONE',  ( 0.000000000000000000, 11.24999999999999467, 0.000000000000000000 ) ) ;
#7826=CIRCLE ( 'NONE', #6929, 2.649999999999999467 ) ;
#7848=FACE_OUTER_BOUND ( 'NONE', #5415, .T. ) ;
#7860=CIRCLE ( 'NONE', #14865, 20.00000000000000000 ) ;
#7874=ORIENTED_EDGE ( 'NONE', *, *, #1771, .T. ) ;
#7887=DIRECTION ( 'NONE',  ( -0.01515971714484241201, 0.000000000000000000, 0.9998850848853023665 ) ) ;
#7891=ADVANCED_FACE ( 'NONE', ( #10400 ), #3080, .F. ) ;
#7905=EDGE_CURVE ( 'NONE', #10656, #6965, #14974, .T. ) ;
#7923=CARTESIAN_POINT ( 'NONE',  ( 0.000000000000000000, 13.24999999999999822, 0.000000000000000000 ) ) ;
#7935=ORIENTED_EDGE ( 'NONE', *, *, #4365, .F. ) ;
#7938=DIRECTION ( 'NONE',  ( -0.000000000000000000, 1.000000000000000000, -0.000000000000000000 ) ) ;
#7955=ORIENTED_EDGE ( 'NONE', *, *, #13718, .F. ) ;
#7956=AXIS2_PLACEMENT_3D ( 'NONE', #9238, #14768, #1822 ) ;
#7993=ORIENTED_EDGE ( 'NONE', *, *, #1787, .F. ) ;
#8016=CARTESIAN_POINT ( 'NONE',  ( 32.50000000000000000, -30.00000000000000000, -2.649999999999631317 ) ) ;
#8017=AXIS2_PLACEMENT_3D ( 'NONE', #12801, #14324, #9934 ) ;
#8029=DIRECTION ( 'NONE',  ( 0.000000000000000000, 0.000000000000000000, 1.000000000000000000 ) ) ;
#8033=EDGE_LOOP ( 'NONE', ( #15335, #8823 ) ) ;
#8047=PRODUCT_DEFINITION ( 'UNKNOWN', '', #16897, #2541 ) ;
#8054=CARTESIAN_POINT ( 'NONE',  ( 0.000000000000000000, 11.24999999999999467, 0.000000000000000000 ) ) ;
#8070=DIRECTION ( 'NONE',  ( 0.000000000000000000, -0.000000000000000000, 1.000000000000000000 ) ) ;
#8142=CIRCLE ( 'NONE', #11495, 2.649999999999995914 ) ;
#8148=EDGE_CURVE ( 'NONE', #18105, #1178, #12390, .T. ) ;
#8151=CARTESIAN_POINT ( 'NONE',  ( 0.000000000000000000, -26.50000000000000000, 0.000000000000000000 ) ) ;
#8168=AXIS2_PLACEMENT_3D ( 'NONE', #10202, #13162, #12790 ) ;
#8176=CARTESIAN_POINT ( 'NONE',  ( 0.000000000000000000, -26.50000000000000000, 25.00000000000000000 ) ) ;
#8180=CARTESIAN_POINT ( 'NONE',  ( 0.000000000000000000, -30.00000000000000000, 25.00000000000000000 ) ) ;
#8268=CIRCLE ( 'NONE', #12835, 23.50000000000001066 ) ;
#8299=DIRECTION ( 'NONE',  ( 0.04803802292983955224, 0.000000000000000000, -0.9988455077503187729 ) ) ;
#8311=ORIENTED_EDGE ( 'NONE', *, *, #14187, .F. ) ;
#8336=DIRECTION ( 'NONE',  ( -0.000000000000000000, 1.000000000000000000, -0.000000000000000000 ) ) ;
#8349=ORIENTED_EDGE ( 'NONE', *, *, #8644, .T. ) ;
#8352=CARTESIAN_POINT ( 'NONE',  ( 32.50000000000000000, -30.00000000000000000, 2.650000000000367617 ) ) ;
#8361=DIRECTION ( 'NONE',  ( 0.9988455077503188839, 0.000000000000000000, 0.04803802292983956612 ) ) ;
#8383=EDGE_CURVE ( 'NONE', #2692, #2531, #16386, .T. ) ;
#8384=VECTOR ( 'NONE', #4199, 1000.000000000000000 ) ;
#8390=FACE_OUTER_BOUND ( 'NONE', #16147, .T. ) ;
#8416=AXIS2_PLACEMENT_3D ( 'NONE', #6591, #12402, #18214 ) ;
#8455=CIRCLE ( 'NONE', #14838, 23.50000000000001066 ) ;
#8466=EDGE_LOOP ( 'NONE', ( #9781, #12506 ) ) ;
#8480=FACE_OUTER_BOUND ( 'NONE', #7397, .T. ) ;
#8486=ORIENTED_EDGE ( 'NONE', *, *, #5992, .F. ) ;
#8488=CARTESIAN_POINT ( 'NONE',  ( 0.000000000000000000, 11.24999999999999645, 25.00000000000000000 ) ) ;
#8508=ORIENTED_EDGE ( 'NONE', *, *, #10959, .F. ) ;
#8532=( GEOMETRIC_REPRESENTATION_CONTEXT ( 3 ) GLOBAL_UNCERTAINTY_ASSIGNED_CONTEXT ( ( #13963 ) ) GLOBAL_UNIT_ASSIGNED_CONTEXT ( ( #4785, #10596, #3458 ) ) REPRESENTATION_CONTEXT ( 'NONE', 'WORKASPACE' ) );
#8572=LINE ( 'NONE', #18378, #12345 ) ;
#8577=ORIENTED_EDGE ( 'NONE', *, *, #15893, .F. ) ;
#8582=VERTEX_POINT ( 'NONE', #13997 ) ;
#8615=ORIENTED_EDGE ( 'NONE', *, *, #14737, .T. ) ;
#8621=ORIENTED_EDGE ( 'NONE', *, *, #16561, .F. ) ;
#8624=DIRECTION ( 'NONE',  ( 0.000000000000000000, 0.000000000000000000, -1.000000000000000000 ) ) ;
#8642=DIRECTION ( 'NONE',  ( 0.000000000000000000, 0.000000000000000000, 1.000000000000000000 ) ) ;
#8643=EDGE_CURVE ( 'NONE', #243, #16476, #5456, .T. ) ;
#8644=EDGE_CURVE ( 'NONE', #17183, #9889, #12762, .T. ) ;
#8653=CARTESIAN_POINT ( 'NONE',  ( 3.061616997868383043E-15, -30.00000000000000000, -25.00000000000000000 ) ) ;
#8655=CARTESIAN_POINT ( 'NONE',  ( 10.04305231718579705, -26.50000000000000000, 33.55933677959249195 ) ) ;
#8661=VERTEX_POINT ( 'NONE', #14447 ) ;
#8669=CIRCLE ( 'NONE', #12627, 25.00000000000000000 ) ;
#8689=ORIENTED_EDGE ( 'NONE', *, *, #3264, .F. ) ;
#8705=VERTEX_POINT ( 'NONE', #12657 ) ;
#8745=DIRECTION ( 'NONE',  ( 0.000000000000000000, 1.000000000000000000, 0.000000000000000000 ) ) ;
#8755=EDGE_CURVE ( 'NONE', #10475, #2531, #3935, .T. ) ;
#8769=CIRCLE ( 'NONE', #2452, 20.00000000000000000 ) ;
#8772=DIRECTION ( 'NONE',  ( -0.000000000000000000, -1.000000000000000000, -0.000000000000000000 ) ) ;
#8796=DIRECTION ( 'NONE',  ( 0.000000000000000000, 0.000000000000000000, 1.000000000000000000 ) ) ;
#8804=DIRECTION ( 'NONE',  ( 0.000000000000000000, 1.000000000000000000, 0.000000000000000000 ) ) ;
#8806=DIRECTION ( 'NONE',  ( 0.000000000000000000, 0.000000000000000000, 1.000000000000000000 ) ) ;
#8822=VERTEX_POINT ( 'NONE', #8834 ) ;
#8823=ORIENTED_EDGE ( 'NONE', *, *, #5164, .F. ) ;
#8828=EDGE_LOOP ( 'NONE', ( #10147, #1044 ) ) ;
#8834=CARTESIAN_POINT ( 'NONE',  ( -26.29305231718584324, -26.50000000000000000, 16.45302069950530566 ) ) ;
#8836=ORIENTED_EDGE ( 'NONE', *, *, #8986, .T. ) ;
#8842=ORIENTED_EDGE ( 'NONE', *, *, #13220, .T. ) ;
#8870=( LENGTH_UNIT ( ) NAMED_UNIT ( * ) SI_UNIT ( .MILLI., .METRE. ) );
#8908=VERTEX_POINT ( 'NONE', #15302 ) ;
#8923=DIRECTION ( 'NONE',  ( -0.000000000000000000, -1.000000000000000000, 0.000000000000000000 ) ) ;
#8929=ORIENTED_EDGE ( 'NONE', *, *, #8755, .F. ) ;
#8964=CARTESIAN_POINT ( 'NONE',  ( 0.000000000000000000, -17.25000000000000355, 27.50000000000000000 ) ) ;
#8969=CARTESIAN_POINT ( 'NONE',  ( 32.50000000000000000, -26.50000000000000000, 3.680389326632394941E-13 ) ) ;
#8978=CIRCLE ( 'NONE', #786, 25.00000000000000000 ) ;
#8986=EDGE_CURVE ( 'NONE', #8661, #9272, #2161, .T. ) ;
#9042=CIRCLE ( 'NONE', #18776, 23.50000000000001066 ) ;
#9050=FACE_BOUND ( 'NONE', #11713, .T. ) ;
#9075=DIRECTION ( 'NONE',  ( -0.000000000000000000, -1.000000000000000000, 0.000000000000000000 ) ) ;
#9077=CIRCLE ( 'NONE', #4517, 2.649999999999999467 ) ;
#9084=DIRECTION ( 'NONE',  ( 0.000000000000000000, 0.000000000000000000, 1.000000000000000000 ) ) ;
#9103=ORIENTED_EDGE ( 'NONE', *, *, #3601, .F. ) ;
#9125=DIRECTION ( 'NONE',  ( -0.9998850848853023665, 0.000000000000000000, -0.01515971714484241721 ) ) ;
#9152=ORIENTED_EDGE ( 'NONE', *, *, #12481, .F. ) ;
#9166=CARTESIAN_POINT ( 'NONE',  ( 32.50000000000000000, -26.50000000000000000, 3.680389326632394941E-13 ) ) ;
#9186=DIRECTION ( 'NONE',  ( -0.000000000000000000, 1.000000000000000000, -0.000000000000000000 ) ) ;
#9206=ORIENTED_EDGE ( 'NONE', *, *, #16809, .T. ) ;
#9216=FACE_OUTER_BOUND ( 'NONE', #4893, .T. ) ;
#9218=VERTEX_POINT ( 'NONE', #8016 ) ;
#9237=DIRECTION ( 'NONE',  ( 0.000000000000000000, 1.000000000000000000, 0.000000000000000000 ) ) ;
#9238=CARTESIAN_POINT ( 'NONE',  ( 10.04305231718605285, -26.50000000000000000, -30.90933677959240811 ) ) ;
#9245=ORIENTED_EDGE ( 'NONE', *, *, #8383, .F. ) ;
#9262=ORIENTED_EDGE ( 'NONE', *, *, #16405, .T. ) ;
#9272=VERTEX_POINT ( 'NONE', #2230 ) ;
#9277=FACE_OUTER_BOUND ( 'NONE', #5756, .T. ) ;
#9290=LINE ( 'NONE', #6066, #18418 ) ;
#9295=ADVANCED_FACE ( 'NONE', ( #4905 ), #13846, .T. ) ;
#9318=AXIS2_PLACEMENT_3D ( 'NONE', #13721, #5139, #2277 ) ;
#9376=AXIS2_PLACEMENT_3D ( 'NONE', #7809, #9237, #16399 ) ;
#9377=PRODUCT ( 'stationary ring', 'stationary ring', '', ( #18698 ) ) ;
#9410=EDGE_LOOP ( 'NONE', ( #18457, #14770, #6298, #8508 ) ) ;
#9414=FACE_BOUND ( 'NONE', #7166, .T. ) ;
#9439=VERTEX_POINT ( 'NONE', #14417 ) ;
#9471=EDGE_CURVE ( 'NONE', #4068, #12311, #12522, .T. ) ;
#9476=LINE ( 'NONE', #13958, #11288 ) ;
#9498=DIRECTION ( 'NONE',  ( -0.000000000000000000, 1.000000000000000000, -0.000000000000000000 ) ) ;
#9505=FACE_BOUND ( 'NONE', #8828, .T. ) ;
#9509=AXIS2_PLACEMENT_3D ( 'NONE', #12080, #15232, #368 ) ;
#9518=CYLINDRICAL_SURFACE ( 'NONE', #18449, 25.00000000000000000 ) ;
#9520=CARTESIAN_POINT ( 'NONE',  ( 32.50000000000000000, -26.50000000000000000, 2.650000000000367617 ) ) ;
#9574=FACE_OUTER_BOUND ( 'NONE', #16630, .T. ) ;
#9575=EDGE_CURVE ( 'NONE', #2531, #10475, #1233, .T. ) ;
#9597=AXIS2_PLACEMENT_3D ( 'NONE', #8054, #13861, #836 ) ;
#9598=ORIENTED_EDGE ( 'NONE', *, *, #4131, .F. ) ;
#9600=ORIENTED_EDGE ( 'NONE', *, *, #9711, .F. ) ;
#9666=DIRECTION ( 'NONE',  ( 1.000000000000000000, 0.000000000000000000, 0.000000000000000000 ) ) ;
#9685=VECTOR ( 'NONE', #3615, 1000.000000000000000 ) ;
#9701=MANIFOLD_SOLID_BREP ( 'M5 Clearance Hole2', #1011 ) ;
#9711=EDGE_CURVE ( 'NONE', #11347, #8582, #13553, .T. ) ;
#9724=LINE ( 'NONE', #12956, #1371 ) ;
#9732=VECTOR ( 'NONE', #4836, 1000.000000000000000 ) ;
#9749=VERTEX_POINT ( 'NONE', #790 ) ;
#9758=APPLICATION_CONTEXT ( 'automotive_design' ) ;
#9773=DIRECTION ( 'NONE',  ( 0.000000000000000000, 1.000000000000000000, 0.000000000000000000 ) ) ;
#9781=ORIENTED_EDGE ( 'NONE', *, *, #14953, .T. ) ;
#9794=VERTEX_POINT ( 'NONE', #1269 ) ;
#9813=CIRCLE ( 'NONE', #3126, 41.00000000000000000 ) ;
#9825=ADVANCED_FACE ( 'NONE', ( #14213 ), #1071, .T. ) ;
#9827=EDGE_LOOP ( 'NONE', ( #3248, #9206 ) ) ;
#9836=CARTESIAN_POINT ( 'NONE',  ( 0.000000000000000000, 11.24999999999999467, 0.000000000000000000 ) ) ;
#9851=MECHANICAL_DESIGN_GEOMETRIC_PRESENTATION_REPRESENTATION('',(#14113),#12278);
#9889=VERTEX_POINT ( 'NONE', #300 ) ;
#9904=CARTESIAN_POINT ( 'NONE',  ( 5.021051876504148963E-15, -30.00000000000000000, 41.00000000000000000 ) ) ;
#9934=DIRECTION ( 'NONE',  ( 1.000000000000000000, 0.000000000000000000, 0.000000000000000000 ) ) ;
#9937=AXIS2_PLACEMENT_3D ( 'NONE', #7923, #3829, #13740 ) ;
#10000=CARTESIAN_POINT ( 'NONE',  ( 0.000000000000000000, -13.75000000000000355, 0.000000000000000000 ) ) ;
#10014=ORIENTED_EDGE ( 'NONE', *, *, #6952, .T. ) ;
#10064=CARTESIAN_POINT ( 'NONE',  ( 0.000000000000000000, -26.50000000000000000, 0.000000000000000000 ) ) ;
#10090=CARTESIAN_POINT ( 'NONE',  ( 10.04305231718579705, -30.00000000000000000, 28.25933677959249835 ) ) ;
#10112=CARTESIAN_POINT ( 'NONE',  ( 0.000000000000000000, -26.50000000000000000, 0.000000000000000000 ) ) ;
#10117=FACE_BOUND ( 'NONE', #6077, .T. ) ;
#10122=DIRECTION ( 'NONE',  ( 0.000000000000000000, 1.000000000000000000, 0.000000000000000000 ) ) ;
#10147=ORIENTED_EDGE ( 'NONE', *, *, #4100, .F. ) ;
#10202=CARTESIAN_POINT ( 'NONE',  ( 0.000000000000000000, -13.75000000000000533, 0.000000000000000000 ) ) ;
#10226=AXIS2_PLACEMENT_3D ( 'NONE', #4493, #10388, #14587 ) ;
#10245=DIRECTION ( 'NONE',  ( -0.000000000000000000, 1.000000000000000000, -0.000000000000000000 ) ) ;
#10261=CIRCLE ( 'NONE', #12701, 2.649999999999999467 ) ;
#10268=AXIS2_PLACEMENT_3D ( 'NONE', #3185, #333, #9084 ) ;
#10272=VERTEX_POINT ( 'NONE', #7389 ) ;
#10315=DIRECTION ( 'NONE',  ( 0.000000000000000000, 0.000000000000000000, 1.000000000000000000 ) ) ;
#10324=CIRCLE ( 'NONE', #11842, 2.649999999999995914 ) ;
#10333=CARTESIAN_POINT ( 'NONE',  ( 0.000000000000000000, -26.50000000000000000, 0.000000000000000000 ) ) ;
#10349=AXIS2_PLACEMENT_3D ( 'NONE', #16314, #9075, #7643 ) ;
#10382=AXIS2_PLACEMENT_3D ( 'NONE', #1008, #6808, #6903 ) ;
#10388=DIRECTION ( 'NONE',  ( 0.000000000000000000, 1.000000000000000000, 0.000000000000000000 ) ) ;
#10400=FACE_OUTER_BOUND ( 'NONE', #1133, .T. ) ;
#10421=ORIENTED_EDGE ( 'NONE', *, *, #14588, .F. ) ;
#10436=FACE_OUTER_BOUND ( 'NONE', #13593, .T. ) ;
#10447=EDGE_CURVE ( 'NONE', #12652, #645, #9476, .T. ) ;
#10475=VERTEX_POINT ( 'NONE', #12235 ) ;
#10498=CARTESIAN_POINT ( 'NONE',  ( 0.000000000000000000, -17.25000000000000355, 25.00000000000000000 ) ) ;
#10502=CARTESIAN_POINT ( 'NONE',  ( 0.000000000000000000, -17.25000000000000355, 0.000000000000000000 ) ) ;
#10517=VECTOR ( 'NONE', #8299, 1000.000000000000000 ) ;
#10549=CIRCLE ( 'NONE', #7802, 25.00000000000000000 ) ;
#10551=FACE_OUTER_BOUND ( 'NONE', #17550, .T. ) ;
#10556=CARTESIAN_POINT ( 'NONE',  ( -26.29305231718584324, -26.50000000000000000, 19.10302069950530779 ) ) ;
#10584=PRODUCT_DEFINITION_SHAPE ( 'NONE', 'NONE',  #8047 ) ;
#10596=( NAMED_UNIT ( * ) PLANE_ANGLE_UNIT ( ) SI_UNIT ( $, .RADIAN. ) );
#10628=EDGE_CURVE ( 'NONE', #14866, #9218, #2163, .T. ) ;
#10631=AXIS2_PLACEMENT_3D ( 'NONE', #6179, #13430, #288 ) ;
#10637=ORIENTED_EDGE ( 'NONE', *, *, #8986, .F. ) ;
#10648=CARTESIAN_POINT ( 'NONE',  ( 0.000000000000000000, 15.00000000000000000, 0.000000000000000000 ) ) ;
#10656=VERTEX_POINT ( 'NONE', #17107 ) ;
#10671=CARTESIAN_POINT ( 'NONE',  ( -23.48826165280196321, 11.24999999999999467, -0.7426739052322690604 ) ) ;
#10737=CIRCLE ( 'NONE', #5275, 25.00000000000000000 ) ;
#10759=VERTEX_POINT ( 'NONE', #2895 ) ;
#10796=VECTOR ( 'NONE', #16257, 1000.000000000000000 ) ;
#10797=CARTESIAN_POINT ( 'NONE',  ( 10.04305231718579705, -26.50000000000000000, 30.90933677959249337 ) ) ;
#10811=ORIENTED_EDGE ( 'NONE', *, *, #295, .T. ) ;
#10819=ORIENTED_EDGE ( 'NONE', *, *, #283, .F. ) ;
#10832=EDGE_CURVE ( 'NONE', #17331, #16237, #3059, .T. ) ;
#10837=DIRECTION ( 'NONE',  ( 0.000000000000000000, 0.000000000000000000, 1.000000000000000000 ) ) ;
#10868=CIRCLE ( 'NONE', #10268, 27.50000000000000000 ) ;
#10924=FACE_OUTER_BOUND ( 'NONE', #614, .T. ) ;
#10925=CARTESIAN_POINT ( 'NONE',  ( -26.29305231718584324, -30.00000000000000000, 19.10302069950530779 ) ) ;
#10945=CARTESIAN_POINT ( 'NONE',  ( 2.449293598294706513E-15, -30.00000000000000000, -20.00000000000000000 ) ) ;
#10954=DIRECTION ( 'NONE',  ( -0.000000000000000000, 1.000000000000000000, -0.000000000000000000 ) ) ;
#10959=EDGE_CURVE ( 'NONE', #14866, #16034, #1929, .T. ) ;
#10961=ORIENTED_EDGE ( 'NONE', *, *, #12813, .T. ) ;
#10978=ORIENTED_EDGE ( 'NONE', *, *, #2549, .F. ) ;
#11003=ORIENTED_EDGE ( 'NONE', *, *, #11721, .F. ) ;
#11038=LINE ( 'NONE', #10945, #6963 ) ;
#11043=CARTESIAN_POINT ( 'NONE',  ( 3.061616997868383043E-15, 15.00000000000000000, -25.00000000000000000 ) ) ;
#11065=DIRECTION ( 'NONE',  ( 0.000000000000000000, 0.000000000000000000, 1.000000000000000000 ) ) ;
#11095=DIRECTION ( 'NONE',  ( 0.000000000000000000, 0.000000000000000000, 1.000000000000000000 ) ) ;
#11111=CARTESIAN_POINT ( 'NONE',  ( -0.3562533529037968383, 11.24999999999999467, 23.49729949480461499 ) ) ;
#11116=CARTESIAN_POINT ( 'NONE',  ( 10.04305231718605285, -30.00000000000000000, -28.25933677959240953 ) ) ;
#11182=VECTOR ( 'NONE', #14115, 1000.000000000000000 ) ;
#11190=ORIENTED_EDGE ( 'NONE', *, *, #6989, .F. ) ;
#11234=ADVANCED_FACE ( 'NONE', ( #10117, #7341, #9050, #1819, #14489, #15924, #11639 ), #13250, .F. ) ;
#11241=LINE ( 'NONE', #8653, #8384 ) ;
#11256=ORIENTED_EDGE ( 'NONE', *, *, #16856, .F. ) ;
#11264=AXIS2_PLACEMENT_3D ( 'NONE', #15550, #6978, #5348 ) ;
#11273=CARTESIAN_POINT ( 'NONE',  ( 10.04305231718579705, -30.00000000000000000, 30.90933677959249337 ) ) ;
#11288=VECTOR ( 'NONE', #15483, 1000.000000000000000 ) ;
#11291=DIRECTION ( 'NONE',  ( 0.000000000000000000, 1.000000000000000000, 0.000000000000000000 ) ) ;
#11347=VERTEX_POINT ( 'NONE', #17809 ) ;
#11350=EDGE_CURVE ( 'NONE', #8822, #12311, #12061, .T. ) ;
#11362=AXIS2_PLACEMENT_3D ( 'NONE', #11273, #5474, #4044 ) ;
#11409=CARTESIAN_POINT ( 'NONE',  ( -23.48826165280197031, 11.24999999999999467, -0.7426739052322692825 ) ) ;
#11437=CIRCLE ( 'NONE', #3823, 25.00000000000000000 ) ;
#11469=DIRECTION ( 'NONE',  ( 0.000000000000000000, 1.000000000000000000, 0.000000000000000000 ) ) ;
#11495=AXIS2_PLACEMENT_3D ( 'NONE', #5465, #13937, #6700 ) ;
#11568=ADVANCED_FACE ( 'NONE', ( #8480 ), #15531, .F. ) ;
#11604=CARTESIAN_POINT ( 'NONE',  ( 32.50000000000000000, -26.50000000000000000, 3.680389326632394941E-13 ) ) ;
#11606=ORIENTED_EDGE ( 'NONE', *, *, #4817, .T. ) ;
#11608=ORIENTED_EDGE ( 'NONE', *, *, #7642, .F. ) ;
#11624=ORIENTED_EDGE ( 'NONE', *, *, #9711, .T. ) ;
#11639=FACE_OUTER_BOUND ( 'NONE', #9827, .T. ) ;
#11689=ADVANCED_FACE ( 'NONE', ( #14657 ), #5985, .F. ) ;
#11713=EDGE_LOOP ( 'NONE', ( #13988, #2647 ) ) ;
#11721=EDGE_CURVE ( 'NONE', #16237, #3613, #13513, .T. ) ;
#11740=CIRCLE ( 'NONE', #6264, 27.50000000000000000 ) ;
#11743=ORIENTED_EDGE ( 'NONE', *, *, #4591, .T. ) ;
#11748=CIRCLE ( 'NONE', #3543, 25.00000000000000000 ) ;
#11765=PLANE ( 'NONE',  #995 ) ;
#11782=VECTOR ( 'NONE', #458, 1000.000000000000000 ) ;
#11842=AXIS2_PLACEMENT_3D ( 'NONE', #15726, #1430, #2677 ) ;
#11918=ADVANCED_FACE ( 'NONE', ( #12749 ), #15601, .F. ) ;
#11929=LINE ( 'NONE', #8964, #18139 ) ;
#11949=ORIENTED_EDGE ( 'NONE', *, *, #7905, .T. ) ;
#11954=AXIS2_PLACEMENT_3D ( 'NONE', #6183, #7617, #470 ) ;
#11977=CARTESIAN_POINT ( 'NONE',  ( -0.3562533529037968383, 11.24999999999999467, 23.49729949480461499 ) ) ;
#11999=DIRECTION ( 'NONE',  ( 0.000000000000000000, -1.000000000000000000, 0.000000000000000000 ) ) ;
#12028=DIRECTION ( 'NONE',  ( -0.000000000000000000, 1.000000000000000000, -0.000000000000000000 ) ) ;
#12061=CIRCLE ( 'NONE', #14811, 2.649999999999999467 ) ;
#12080=CARTESIAN_POINT ( 'NONE',  ( 0.000000000000000000, -26.50000000000000000, 0.000000000000000000 ) ) ;
#12115=ORIENTED_EDGE ( 'NONE', *, *, #6426, .F. ) ;
#12125=ORIENTED_EDGE ( 'NONE', *, *, #3429, .F. ) ;
#12129=LINE ( 'NONE', #12221, #10517 ) ;
#12177=CARTESIAN_POINT ( 'NONE',  ( -0.3562533529037968383, 13.24999999999999467, 23.49729949480461499 ) ) ;
#12190=ORIENTED_EDGE ( 'NONE', *, *, #13445, .F. ) ;
#12221=CARTESIAN_POINT ( 'NONE',  ( -1.128893538851230005, 11.24999999999999467, 23.47286943213250154 ) ) ;
#12235=CARTESIAN_POINT ( 'NONE',  ( 10.04305231718605285, -26.50000000000000000, -33.55933677959240669 ) ) ;
#12268=DIRECTION ( 'NONE',  ( 0.000000000000000000, 1.000000000000000000, 0.000000000000000000 ) ) ;
#12278=( GEOMETRIC_REPRESENTATION_CONTEXT ( 3 ) GLOBAL_UNCERTAINTY_ASSIGNED_CONTEXT ( ( #3680 ) ) GLOBAL_UNIT_ASSIGNED_CONTEXT ( ( #8870, #16493, #3449 ) ) REPRESENTATION_CONTEXT ( 'NONE', 'WORKASPACE' ) );
#12310=FACE_OUTER_BOUND ( 'NONE', #12476, .T. ) ;
#12311=VERTEX_POINT ( 'NONE', #18397 ) ;
#12345=VECTOR ( 'NONE', #15535, 1000.000000000000000 ) ;
#12390=LINE ( 'NONE', #18203, #2074 ) ;
#12402=DIRECTION ( 'NONE',  ( 0.000000000000000000, -1.000000000000000000, 0.000000000000000000 ) ) ;
#12410=ORIENTED_EDGE ( 'NONE', *, *, #16856, .T. ) ;
#12418=CARTESIAN_POINT ( 'NONE',  ( -26.29305231718568336, -26.50000000000000000, -16.45302069950552237 ) ) ;
#12448=CARTESIAN_POINT ( 'NONE',  ( 0.000000000000000000, -30.00000000000000000, 20.00000000000000000 ) ) ;
#12473=AXIS2_PLACEMENT_3D ( 'NONE', #4157, #13009, #8806 ) ;
#12476=EDGE_LOOP ( 'NONE', ( #403, #14777, #17371, #17114 ) ) ;
#12481=EDGE_CURVE ( 'NONE', #4230, #7648, #13249, .T. ) ;
#12506=ORIENTED_EDGE ( 'NONE', *, *, #12481, .T. ) ;
#12511=DIRECTION ( 'NONE',  ( -0.000000000000000000, -1.000000000000000000, 0.000000000000000000 ) ) ;
#12519=ORIENTED_EDGE ( 'NONE', *, *, #16809, .F. ) ;
#12522=LINE ( 'NONE', #5376, #1534 ) ;
#12566=AXIS2_PLACEMENT_3D ( 'NONE', #6813, #1208, #7007 ) ;
#12568=DIRECTION ( 'NONE',  ( 1.000000000000000000, 0.000000000000000000, 0.000000000000000000 ) ) ;
#12569=CIRCLE ( 'NONE', #11954, 25.00000000000000000 ) ;
#12602=LINE ( 'NONE', #12418, #17530 ) ;
#12605=ORIENTED_EDGE ( 'NONE', *, *, #10832, .T. ) ;
#12627=AXIS2_PLACEMENT_3D ( 'NONE', #10648, #8745, #13226 ) ;
#12648=LINE ( 'NONE', #8180, #9685 ) ;
#12652=VERTEX_POINT ( 'NONE', #6391 ) ;
#12657=CARTESIAN_POINT ( 'NONE',  ( 3.061616997868383043E-15, 13.24999999999999822, -25.00000000000000000 ) ) ;
#12663=ORIENTED_EDGE ( 'NONE', *, *, #1771, .F. ) ;
#12674=VERTEX_POINT ( 'NONE', #11043 ) ;
#12700=EDGE_LOOP ( 'NONE', ( #5975, #16067, #468, #9152 ) ) ;
#12701=AXIS2_PLACEMENT_3D ( 'NONE', #9166, #16705, #3561 ) ;
#12749=FACE_OUTER_BOUND ( 'NONE', #310, .T. ) ;
#12762=LINE ( 'NONE', #11409, #1491 ) ;
#12768=VERTEX_POINT ( 'NONE', #18004 ) ;
#12772=CARTESIAN_POINT ( 'NONE',  ( -26.29305231718568336, -26.50000000000000000, -19.10302069950552095 ) ) ;
#12790=DIRECTION ( 'NONE',  ( 0.000000000000000000, 0.000000000000000000, 1.000000000000000000 ) ) ;
#12801=CARTESIAN_POINT ( 'NONE',  ( 0.000000000000000000, 0.000000000000000000, 0.000000000000000000 ) ) ;
#12813=EDGE_CURVE ( 'NONE', #8705, #12674, #9724, .T. ) ;
#12831=EDGE_CURVE ( 'NONE', #15594, #4230, #8572, .T. ) ;
#12835=AXIS2_PLACEMENT_3D ( 'NONE', #4457, #8923, #17419 ) ;
#12849=DIRECTION ( 'NONE',  ( 0.000000000000000000, 1.000000000000000000, 0.000000000000000000 ) ) ;
#12863=EDGE_LOOP ( 'NONE', ( #13388, #12190, #14068, #13233 ) ) ;
#12910=VERTEX_POINT ( 'NONE', #9904 ) ;
#12940=FACE_OUTER_BOUND ( 'NONE', #7767, .T. ) ;
#12948=CARTESIAN_POINT ( 'NONE',  ( -1.200950573245989306, -30.00000000000000000, 24.97113769375797787 ) ) ;
#12956=CARTESIAN_POINT ( 'NONE',  ( 3.061616997868383043E-15, -30.00000000000000000, -25.00000000000000000 ) ) ;
#12979=ORIENTED_EDGE ( 'NONE', *, *, #11350, .F. ) ;
#13009=DIRECTION ( 'NONE',  ( 0.000000000000000000, 1.000000000000000000, 0.000000000000000000 ) ) ;
#13028=ORIENTED_EDGE ( 'NONE', *, *, #9471, .F. ) ;
#13043=AXIS2_PLACEMENT_3D ( 'NONE', #7689, #12268, #15511 ) ;
#13061=ORIENTED_EDGE ( 'NONE', *, *, #3883, .F. ) ;
#13129=CYLINDRICAL_SURFACE ( 'NONE', #14205, 20.00000000000000000 ) ;
#13140=DIRECTION ( 'NONE',  ( 0.000000000000000000, -0.000000000000000000, 1.000000000000000000 ) ) ;
#13146=FACE_OUTER_BOUND ( 'NONE', #16075, .T. ) ;
#13157=ORIENTED_EDGE ( 'NONE', *, *, #11721, .T. ) ;
#13162=DIRECTION ( 'NONE',  ( -0.000000000000000000, -1.000000000000000000, -0.000000000000000000 ) ) ;
#13174=AXIS2_PLACEMENT_3D ( 'NONE', #11604, #17409, #4361 ) ;
#13176=CIRCLE ( 'NONE', #6162, 23.50000000000001066 ) ;
#13209=ORIENTED_EDGE ( 'NONE', *, *, #1576, .F. ) ;
#13220=EDGE_CURVE ( 'NONE', #72, #13484, #7383, .T. ) ;
#13226=DIRECTION ( 'NONE',  ( 0.000000000000000000, 0.000000000000000000, 1.000000000000000000 ) ) ;
#13233=ORIENTED_EDGE ( 'NONE', *, *, #9575, .T. ) ;
#13238=DIRECTION ( 'NONE',  ( -0.000000000000000000, 1.000000000000000000, -0.000000000000000000 ) ) ;
#13249=CIRCLE ( 'NONE', #17808, 27.50000000000000000 ) ;
#13250=PLANE ( 'NONE',  #10226 ) ;
#13279=DIRECTION ( 'NONE',  ( 0.000000000000000000, 0.000000000000000000, 1.000000000000000000 ) ) ;
#13306=AXIS2_PLACEMENT_3D ( 'NONE', #10556, #2173, #17984 ) ;
#13324=ORIENTED_EDGE ( 'NONE', *, *, #8643, .T. ) ;
#13366=VERTEX_POINT ( 'NONE', #18061 ) ;
#13388=ORIENTED_EDGE ( 'NONE', *, *, #13606, .F. ) ;
#13405=ORIENTED_EDGE ( 'NONE', *, *, #18657, .F. ) ;
#13411=DIRECTION ( 'NONE',  ( -0.000000000000000000, 1.000000000000000000, -0.000000000000000000 ) ) ;
#13427=FACE_BOUND ( 'NONE', #4404, .T. ) ;
#13430=DIRECTION ( 'NONE',  ( -0.000000000000000000, 1.000000000000000000, -0.000000000000000000 ) ) ;
#13445=EDGE_CURVE ( 'NONE', #2692, #6586, #5637, .T. ) ;
#13484=VERTEX_POINT ( 'NONE', #18545 ) ;
#13502=EDGE_LOOP ( 'NONE', ( #4618, #7874 ) ) ;
#13508=ORIENTED_EDGE ( 'NONE', *, *, #13934, .T. ) ;
#13513=LINE ( 'NONE', #11977, #11782 ) ;
#13517=ORIENTED_EDGE ( 'NONE', *, *, #1291, .F. ) ;
#13526=ORIENTED_EDGE ( 'NONE', *, *, #14737, .F. ) ;
#13529=DIRECTION ( 'NONE',  ( -0.000000000000000000, 1.000000000000000000, -0.000000000000000000 ) ) ;
#13541=( NAMED_UNIT ( * ) SI_UNIT ( $, .STERADIAN. ) SOLID_ANGLE_UNIT ( ) );
#13553=LINE ( 'NONE', #18110, #17060 ) ;
#13563=FACE_OUTER_BOUND ( 'NONE', #14998, .T. ) ;
#13569=VERTEX_POINT ( 'NONE', #1492 ) ;
#13581=AXIS2_PLACEMENT_3D ( 'NONE', #10112, #15834, #4308 ) ;
#13593=EDGE_LOOP ( 'NONE', ( #14443, #10978, #8836, #1314 ) ) ;
#13606=EDGE_CURVE ( 'NONE', #6586, #10475, #15785, .T. ) ;
#13684=ORIENTED_EDGE ( 'NONE', *, *, #14352, .T. ) ;
#13688=CARTESIAN_POINT ( 'NONE',  ( 2.449293598294706513E-15, -30.00000000000000000, -20.00000000000000000 ) ) ;
#13693=AXIS2_PLACEMENT_3D ( 'NONE', #1739, #14694, #8796 ) ;
#13699=CARTESIAN_POINT ( 'NONE',  ( 0.000000000000000000, -17.25000000000000355, 0.000000000000000000 ) ) ;
#13718=EDGE_CURVE ( 'NONE', #5558, #5435, #8978, .T. ) ;
#13721=CARTESIAN_POINT ( 'NONE',  ( -26.29305231718568336, -26.50000000000000000, -19.10302069950552095 ) ) ;
#13729=DIRECTION ( 'NONE',  ( -0.000000000000000000, 1.000000000000000000, -0.000000000000000000 ) ) ;
#13740=DIRECTION ( 'NONE',  ( 0.000000000000000000, 0.000000000000000000, 1.000000000000000000 ) ) ;
#13752=ORIENTED_EDGE ( 'NONE', *, *, #10628, .T. ) ;
#13784=ORIENTED_EDGE ( 'NONE', *, *, #3429, .T. ) ;
#13846=CYLINDRICAL_SURFACE ( 'NONE', #5482, 25.00000000000000000 ) ;
#13861=DIRECTION ( 'NONE',  ( 0.000000000000000000, 1.000000000000000000, 0.000000000000000000 ) ) ;
#13879=ORIENTED_EDGE ( 'NONE', *, *, #4834, .F. ) ;
#13880=CARTESIAN_POINT ( 'NONE',  ( 0.000000000000000000, 13.24999999999999467, 0.000000000000000000 ) ) ;
#13881=CARTESIAN_POINT ( 'NONE',  ( 3.061616997868383043E-15, 11.24999999999999645, -25.00000000000000000 ) ) ;
#13884=ORIENTED_EDGE ( 'NONE', *, *, #4028, .F. ) ;
#13909=ORIENTED_EDGE ( 'NONE', *, *, #10628, .F. ) ;
#13925=ORIENTED_EDGE ( 'NONE', *, *, #16227, .T. ) ;
#13934=EDGE_CURVE ( 'NONE', #16268, #8822, #6717, .T. ) ;
#13937=DIRECTION ( 'NONE',  ( 0.000000000000000000, 1.000000000000000000, 0.000000000000000000 ) ) ;
#13938=DIRECTION ( 'NONE',  ( 0.000000000000000000, -1.000000000000000000, 0.000000000000000000 ) ) ;
#13958=CARTESIAN_POINT ( 'NONE',  ( -1.128893538851230005, 13.24999999999999467, 23.47286943213250154 ) ) ;
#13963=UNCERTAINTY_MEASURE_WITH_UNIT (LENGTH_MEASURE( 1.000000000000000082E-05 ), #4785, 'distance_accuracy_value', 'NONE');
#13976=AXIS2_PLACEMENT_3D ( 'NONE', #5314, #16952, #3998 ) ;
#13978=CARTESIAN_POINT ( 'NONE',  ( 10.04305231718605285, -30.00000000000000000, -30.90933677959240811 ) ) ;
#13986=EDGE_LOOP ( 'NONE', ( #11190, #12979 ) ) ;
#13988=ORIENTED_EDGE ( 'NONE', *, *, #16561, .T. ) ;
#13997=CARTESIAN_POINT ( 'NONE',  ( -0.3789929286210603765, 11.24999999999999645, 24.99712712213256438 ) ) ;
#13999=AXIS2_PLACEMENT_3D ( 'NONE', #463, #11291, #17113 ) ;
#14003=CARTESIAN_POINT ( 'NONE',  ( 0.000000000000000000, -30.00000000000000000, 0.000000000000000000 ) ) ;
#14047=CARTESIAN_POINT ( 'NONE',  ( -26.29305231718584324, -26.50000000000000000, 16.45302069950530566 ) ) ;
#14060=CARTESIAN_POINT ( 'NONE',  ( 0.000000000000000000, 13.24999999999999822, 0.000000000000000000 ) ) ;
#14068=ORIENTED_EDGE ( 'NONE', *, *, #8383, .T. ) ;
#14113=STYLED_ITEM ( 'NONE', ( #3079 ), #5356 ) ;
#14115=DIRECTION ( 'NONE',  ( -0.000000000000000000, 1.000000000000000000, -0.000000000000000000 ) ) ;
#14128=EDGE_LOOP ( 'NONE', ( #13209, #15610 ) ) ;
#14131=AXIS2_PLACEMENT_3D ( 'NONE', #5211, #18069, #6651 ) ;
#14187=EDGE_CURVE ( 'NONE', #8908, #9439, #1836, .T. ) ;
#14192=AXIS2_PLACEMENT_3D ( 'NONE', #6061, #6152, #165 ) ;
#14205=AXIS2_PLACEMENT_3D ( 'NONE', #15803, #2754, #4280 ) ;
#14213=FACE_OUTER_BOUND ( 'NONE', #18281, .T. ) ;
#14247=VECTOR ( 'NONE', #4592, 1000.000000000000000 ) ;
#14255=EDGE_CURVE ( 'NONE', #13366, #7648, #11929, .T. ) ;
#14324=DIRECTION ( 'NONE',  ( 0.000000000000000000, 0.000000000000000000, 1.000000000000000000 ) ) ;
#14352=EDGE_CURVE ( 'NONE', #8908, #11347, #819, .T. ) ;
#14373=ORIENTED_EDGE ( 'NONE', *, *, #11350, .T. ) ;
#14417=CARTESIAN_POINT ( 'NONE',  ( 0.000000000000000000, 15.00000000000000000, 25.00000000000000000 ) ) ;
#14422=ORIENTED_EDGE ( 'NONE', *, *, #16405, .F. ) ;
#14432=ORIENTED_EDGE ( 'NONE', *, *, #16410, .F. ) ;
#14436=CARTESIAN_POINT ( 'NONE',  ( 23.48826165280197031, 11.24999999999999467, 0.7426739052322662848 ) ) ;
#14443=ORIENTED_EDGE ( 'NONE', *, *, #15992, .F. ) ;
#14447=CARTESIAN_POINT ( 'NONE',  ( 0.000000000000000000, -30.00000000000000000, 20.00000000000000000 ) ) ;
#14448=EDGE_CURVE ( 'NONE', #72, #17369, #5970, .T. ) ;
#14456=ADVANCED_FACE ( 'NONE', ( #1268 ), #18499, .T. ) ;
#14489=FACE_BOUND ( 'NONE', #3302, .T. ) ;
#14521=ORIENTED_EDGE ( 'NONE', *, *, #6563, .F. ) ;
#14587=DIRECTION ( 'NONE',  ( 0.000000000000000000, -0.000000000000000000, 1.000000000000000000 ) ) ;
#14588=EDGE_CURVE ( 'NONE', #10272, #16476, #2582, .T. ) ;
#14628=CARTESIAN_POINT ( 'NONE',  ( 0.000000000000000000, -26.50000000000000000, -41.00000000000000000 ) ) ;
#14654=PLANE ( 'NONE',  #7142 ) ;
#14657=FACE_OUTER_BOUND ( 'NONE', #7070, .T. ) ;
#14673=AXIS2_PLACEMENT_3D ( 'NONE', #8969, #15080, #2032 ) ;
#14694=DIRECTION ( 'NONE',  ( -0.000000000000000000, 1.000000000000000000, -0.000000000000000000 ) ) ;
#14737=EDGE_CURVE ( 'NONE', #16747, #2351, #10549, .T. ) ;
#14768=DIRECTION ( 'NONE',  ( -0.000000000000000000, 1.000000000000000000, -0.000000000000000000 ) ) ;
#14770=ORIENTED_EDGE ( 'NONE', *, *, #1787, .T. ) ;
#14777=ORIENTED_EDGE ( 'NONE', *, *, #12831, .T. ) ;
#14796=ORIENTED_EDGE ( 'NONE', *, *, #13934, .F. ) ;
#14811=AXIS2_PLACEMENT_3D ( 'NONE', #3635, #13529, #480 ) ;
#14816=DIRECTION ( 'NONE',  ( 0.000000000000000000, 0.000000000000000000, 1.000000000000000000 ) ) ;
#14838=AXIS2_PLACEMENT_3D ( 'NONE', #6609, #12511, #5077 ) ;
#14865=AXIS2_PLACEMENT_3D ( 'NONE', #6504, #3660, #799 ) ;
#14866=VERTEX_POINT ( 'NONE', #8352 ) ;
#14883=DIRECTION ( 'NONE',  ( -0.000000000000000000, 1.000000000000000000, -0.000000000000000000 ) ) ;
#14953=EDGE_CURVE ( 'NONE', #7648, #4230, #18791, .T. ) ;
#14974=LINE ( 'NONE', #4776, #14247 ) ;
#14981=CARTESIAN_POINT ( 'NONE',  ( 0.000000000000000000, -30.00000000000000000, 25.00000000000000000 ) ) ;
#14983=CARTESIAN_POINT ( 'NONE',  ( 3.367778697655221307E-15, -17.25000000000000355, -27.50000000000000000 ) ) ;
#14990=CARTESIAN_POINT ( 'NONE',  ( 0.000000000000000000, -30.00000000000000000, 0.000000000000000000 ) ) ;
#14998=EDGE_LOOP ( 'NONE', ( #3290, #7955, #3770, #8615 ) ) ;
#15002=CARTESIAN_POINT ( 'NONE',  ( -1.128893538851230005, 13.24999999999999467, 23.47286943213250154 ) ) ;
#15046=VECTOR ( 'NONE', #3416, 1000.000000000000000 ) ;
#15060=CARTESIAN_POINT ( 'NONE',  ( -26.29305231718568336, -26.50000000000000000, -16.45302069950552237 ) ) ;
#15069=EDGE_LOOP ( 'NONE', ( #14521, #16010, #8842, #12519 ) ) ;
#15080=DIRECTION ( 'NONE',  ( -0.000000000000000000, 1.000000000000000000, -0.000000000000000000 ) ) ;
#15092=VECTOR ( 'NONE', #17738, 1000.000000000000000 ) ;
#15104=DIRECTION ( 'NONE',  ( 0.000000000000000000, 1.000000000000000000, 0.000000000000000000 ) ) ;
#15158=CYLINDRICAL_SURFACE ( 'NONE', #9376, 23.50000000000001066 ) ;
#15175=ORIENTED_EDGE ( 'NONE', *, *, #18805, .F. ) ;
#15182=ADVANCED_FACE ( 'NONE', ( #9277 ), #7662, .F. ) ;
#15193=DIRECTION ( 'NONE',  ( 0.000000000000000000, 0.000000000000000000, 1.000000000000000000 ) ) ;
#15215=CARTESIAN_POINT ( 'NONE',  ( 0.000000000000000000, -17.25000000000000355, 0.000000000000000000 ) ) ;
#15232=DIRECTION ( 'NONE',  ( 0.000000000000000000, -1.000000000000000000, 0.000000000000000000 ) ) ;
#15282=LINE ( 'NONE', #6807, #1149 ) ;
#15300=EDGE_CURVE ( 'NONE', #18412, #645, #15282, .T. ) ;
#15302=CARTESIAN_POINT ( 'NONE',  ( 0.000000000000000000, 13.24999999999999822, 25.00000000000000000 ) ) ;
#15314=ORIENTED_EDGE ( 'NONE', *, *, #10959, .T. ) ;
#15319=PLANE ( 'NONE',  #9509 ) ;
#15335=ORIENTED_EDGE ( 'NONE', *, *, #6742, .F. ) ;
#15350=FACE_OUTER_BOUND ( 'NONE', #3083, .T. ) ;
#15427=CIRCLE ( 'NONE', #9318, 2.649999999999999467 ) ;
#15439=DIRECTION ( 'NONE',  ( 0.000000000000000000, 1.000000000000000000, 0.000000000000000000 ) ) ;
#15446=CARTESIAN_POINT ( 'NONE',  ( 0.000000000000000000, -26.50000000000000000, -41.00000000000000000 ) ) ;
#15448=AXIS2_PLACEMENT_3D ( 'NONE', #4125, #2695, #2303 ) ;
#15469=DIRECTION ( 'NONE',  ( 0.000000000000000000, 1.000000000000000000, 0.000000000000000000 ) ) ;
#15472=ORIENTED_EDGE ( 'NONE', *, *, #3601, .T. ) ;
#15483=DIRECTION ( 'NONE',  ( 0.04803802292983955224, 0.000000000000000000, -0.9988455077503187729 ) ) ;
#15509=CARTESIAN_POINT ( 'NONE',  ( -1.128893538851230005, 11.24999999999999467, 23.47286943213250154 ) ) ;
#15511=DIRECTION ( 'NONE',  ( 1.000000000000000000, 0.000000000000000000, 0.000000000000000000 ) ) ;
#15531=CYLINDRICAL_SURFACE ( 'NONE', #17548, 2.649999999999999467 ) ;
#15535=DIRECTION ( 'NONE',  ( 0.000000000000000000, 1.000000000000000000, 0.000000000000000000 ) ) ;
#15537=DIRECTION ( 'NONE',  ( 0.000000000000000000, 0.000000000000000000, 1.000000000000000000 ) ) ;
#15550=CARTESIAN_POINT ( 'NONE',  ( 0.000000000000000000, -30.00000000000000000, 0.000000000000000000 ) ) ;
#15553=DIRECTION ( 'NONE',  ( -0.000000000000000000, 1.000000000000000000, -0.000000000000000000 ) ) ;
#15594=VERTEX_POINT ( 'NONE', #14983 ) ;
#15601=PLANE ( 'NONE',  #528 ) ;
#15610=ORIENTED_EDGE ( 'NONE', *, *, #18060, .F. ) ;
#15726=CARTESIAN_POINT ( 'NONE',  ( 10.04305231718579705, -30.00000000000000000, 30.90933677959249337 ) ) ;
#15785=LINE ( 'NONE', #17316, #2294 ) ;
#15803=CARTESIAN_POINT ( 'NONE',  ( 0.000000000000000000, -30.00000000000000000, 0.000000000000000000 ) ) ;
#15806=DIRECTION ( 'NONE',  ( -0.000000000000000000, -1.000000000000000000, -0.000000000000000000 ) ) ;
#15822=ORIENTED_EDGE ( 'NONE', *, *, #295, .F. ) ;
#15823=DIRECTION ( 'NONE',  ( 0.000000000000000000, 1.000000000000000000, 0.000000000000000000 ) ) ;
#15834=DIRECTION ( 'NONE',  ( 0.000000000000000000, -1.000000000000000000, 0.000000000000000000 ) ) ;
#15849=CARTESIAN_POINT ( 'NONE',  ( 0.000000000000000000, -30.00000000000000000, 0.000000000000000000 ) ) ;
#15893=EDGE_CURVE ( 'NONE', #10272, #10656, #1772, .T. ) ;
#15895=CARTESIAN_POINT ( 'NONE',  ( 23.48826165280196321, 11.24999999999999467, 0.7426739052322660628 ) ) ;
#15907=CIRCLE ( 'NONE', #6776, 2.649999999999999467 ) ;
#15924=FACE_BOUND ( 'NONE', #16497, .T. ) ;
#15939=CIRCLE ( 'NONE', #7717, 25.00000000000000000 ) ;
#15972=CARTESIAN_POINT ( 'NONE',  ( -26.29305231718584324, -30.00000000000000000, 19.10302069950530779 ) ) ;
#15992=EDGE_CURVE ( 'NONE', #3056, #10759, #11038, .T. ) ;
#15998=ORIENTED_EDGE ( 'NONE', *, *, #16227, .F. ) ;
#16006=AXIS2_PLACEMENT_3D ( 'NONE', #1212, #7466, #522 ) ;
#16010=ORIENTED_EDGE ( 'NONE', *, *, #5992, .T. ) ;
#16034=VERTEX_POINT ( 'NONE', #9520 ) ;
#16049=VECTOR ( 'NONE', #5596, 1000.000000000000000 ) ;
#16067=ORIENTED_EDGE ( 'NONE', *, *, #3264, .T. ) ;
#16075=EDGE_LOOP ( 'NONE', ( #17473, #2342, #13879, #6589 ) ) ;
#16092=AXIS2_PLACEMENT_3D ( 'NONE', #5428, #15806, #8642 ) ;
#16108=EDGE_CURVE ( 'NONE', #5435, #2351, #11241, .T. ) ;
#16125=SURFACE_STYLE_USAGE ( .BOTH. , #4871 ) ;
#16141=DIRECTION ( 'NONE',  ( 0.000000000000000000, 1.000000000000000000, 0.000000000000000000 ) ) ;
#16147=EDGE_LOOP ( 'NONE', ( #4243, #131, #3202, #11003 ) ) ;
#16227=EDGE_CURVE ( 'NONE', #9439, #12674, #8669, .T. ) ;
#16237=VERTEX_POINT ( 'NONE', #7603 ) ;
#16242=ADVANCED_FACE ( 'NONE', ( #5982, #7321 ), #14654, .T. ) ;
#16257=DIRECTION ( 'NONE',  ( -0.000000000000000000, 1.000000000000000000, -0.000000000000000000 ) ) ;
#16268=VERTEX_POINT ( 'NONE', #4844 ) ;
#16281=AXIS2_PLACEMENT_3D ( 'NONE', #13978, #1123, #2448 ) ;
#16300=ORIENTED_EDGE ( 'NONE', *, *, #15893, .T. ) ;
#16314=CARTESIAN_POINT ( 'NONE',  ( 0.000000000000000000, 11.24999999999999467, 0.000000000000000000 ) ) ;
#16318=VECTOR ( 'NONE', #17083, 1000.000000000000000 ) ;
#16358=EDGE_CURVE ( 'NONE', #4068, #16268, #2274, .T. ) ;
#16364=EDGE_CURVE ( 'NONE', #10759, #9272, #4110, .T. ) ;
#16374=CARTESIAN_POINT ( 'NONE',  ( 3.061616997868383043E-15, -26.50000000000000000, -25.00000000000000000 ) ) ;
#16386=LINE ( 'NONE', #17527, #17007 ) ;
#16399=DIRECTION ( 'NONE',  ( 0.9995004958639132076, 0.000000000000000000, 0.03160314490350067673 ) ) ;
#16402=ORIENTED_EDGE ( 'NONE', *, *, #18411, .F. ) ;
#16405=EDGE_CURVE ( 'NONE', #16237, #8582, #5303, .T. ) ;
#16406=FILL_AREA_STYLE ('',( #3162 ) ) ;
#16410=EDGE_CURVE ( 'NONE', #3613, #11347, #2083, .T. ) ;
#16423=CYLINDRICAL_SURFACE ( 'NONE', #18514, 25.00000000000000000 ) ;
#16446=STYLED_ITEM('',(#18890),#9701);
#16451=CARTESIAN_POINT ( 'NONE',  ( -26.29305231718568336, -26.50000000000000000, -21.75302069950551953 ) ) ;
#16476=VERTEX_POINT ( 'NONE', #13881 ) ;
#16493=( NAMED_UNIT ( * ) PLANE_ANGLE_UNIT ( ) SI_UNIT ( $, .RADIAN. ) );
#16497=EDGE_LOOP ( 'NONE', ( #4627, #4183 ) ) ;
#16505=FACE_OUTER_BOUND ( 'NONE', #9410, .T. ) ;
#16532=ORIENTED_EDGE ( 'NONE', *, *, #4131, .T. ) ;
#16553=FACE_BOUND ( 'NONE', #13986, .T. ) ;
#16561=EDGE_CURVE ( 'NONE', #6386, #13569, #15907, .T. ) ;
#16578=CARTESIAN_POINT ( 'NONE',  ( 10.04305231718579705, -26.50000000000000000, 30.90933677959249337 ) ) ;
#16618=DIRECTION ( 'NONE',  ( 0.000000000000000000, 0.000000000000000000, 1.000000000000000000 ) ) ;
#16629=AXIS2_PLACEMENT_3D ( 'NONE', #7778, #9125, #7408 ) ;
#16630=EDGE_LOOP ( 'NONE', ( #17892, #8689 ) ) ;
#16660=CARTESIAN_POINT ( 'NONE',  ( -0.3562533529037968383, 13.24999999999999467, 23.49729949480461499 ) ) ;
#16663=CARTESIAN_POINT ( 'NONE',  ( -1.200950573245989306, 11.24999999999999645, 24.97113769375797432 ) ) ;
#16669=CIRCLE ( 'NONE', #248, 41.00000000000000000 ) ;
#16671=DIRECTION ( 'NONE',  ( 0.000000000000000000, 1.000000000000000000, 0.000000000000000000 ) ) ;
#16681=ORIENTED_EDGE ( 'NONE', *, *, #13606, .T. ) ;
#16694=ADVANCED_FACE ( 'NONE', ( #16505 ), #6126, .F. ) ;
#16705=DIRECTION ( 'NONE',  ( -0.000000000000000000, 1.000000000000000000, -0.000000000000000000 ) ) ;
#16742=SHAPE_REPRESENTATION ( 'stationary ring', ( #8017 ), #737 ) ;
#16747=VERTEX_POINT ( 'NONE', #10498 ) ;
#16748=CYLINDRICAL_SURFACE ( 'NONE', #17279, 2.649999999999999467 ) ;
#16749=DIRECTION ( 'NONE',  ( 0.000000000000000000, 1.000000000000000000, 0.000000000000000000 ) ) ;
#16755=CARTESIAN_POINT ( 'NONE',  ( 10.04305231718605285, -26.50000000000000000, -30.90933677959240811 ) ) ;
#16809=EDGE_CURVE ( 'NONE', #12910, #13484, #9813, .T. ) ;
#16847=DIRECTION ( 'NONE',  ( -0.000000000000000000, 1.000000000000000000, -0.000000000000000000 ) ) ;
#16856=EDGE_CURVE ( 'NONE', #17183, #17331, #13176, .T. ) ;
#16867=DIRECTION ( 'NONE',  ( 0.000000000000000000, 0.000000000000000000, 1.000000000000000000 ) ) ;
#16882=VECTOR ( 'NONE', #7887, 1000.000000000000000 ) ;
#16897=PRODUCT_DEFINITION_FORMATION_WITH_SPECIFIED_SOURCE ( 'ANY', '', #9377, .NOT_KNOWN. ) ;
#16908=DIRECTION ( 'NONE',  ( 0.000000000000000000, -1.000000000000000000, 0.000000000000000000 ) ) ;
#16919=DIRECTION ( 'NONE',  ( 0.000000000000000000, -0.000000000000000000, 1.000000000000000000 ) ) ;
#16952=DIRECTION ( 'NONE',  ( -0.000000000000000000, 1.000000000000000000, -0.000000000000000000 ) ) ;
#16993=LINE ( 'NONE', #3944, #11182 ) ;
#17007=VECTOR ( 'NONE', #13238, 1000.000000000000000 ) ;
#17011=AXIS2_PLACEMENT_3D ( 'NONE', #16755, #16847, #18074 ) ;
#17039=AXIS2_PLACEMENT_3D ( 'NONE', #5540, #15823, #1163 ) ;
#17060=VECTOR ( 'NONE', #6309, 1000.000000000000000 ) ;
#17083=DIRECTION ( 'NONE',  ( 0.000000000000000000, 1.000000000000000000, 0.000000000000000000 ) ) ;
#17091=EDGE_LOOP ( 'NONE', ( #13925, #5130 ) ) ;
#17107=CARTESIAN_POINT ( 'NONE',  ( 0.000000000000000000, -13.75000000000000533, 25.00000000000000000 ) ) ;
#17113=DIRECTION ( 'NONE',  ( 0.000000000000000000, 0.000000000000000000, 1.000000000000000000 ) ) ;
#17114=ORIENTED_EDGE ( 'NONE', *, *, #14255, .F. ) ;
#17115=ORIENTED_EDGE ( 'NONE', *, *, #3883, .T. ) ;
#17157=CYLINDRICAL_SURFACE ( 'NONE', #17039, 23.50000000000001066 ) ;
#17179=EDGE_LOOP ( 'NONE', ( #6069, #330, #6505, #631 ) ) ;
#17183=VERTEX_POINT ( 'NONE', #10671 ) ;
#17222=ADVANCED_FACE ( 'NONE', ( #4585 ), #3444, .F. ) ;
#17225=AXIS2_PLACEMENT_3D ( 'NONE', #15215, #9773, #16919 ) ;
#17247=PLANE ( 'NONE',  #1741 ) ;
#17268=CIRCLE ( 'NONE', #5996, 2.649999999999995914 ) ;
#17279=AXIS2_PLACEMENT_3D ( 'NONE', #3699, #9498, #849 ) ;
#17282=EDGE_CURVE ( 'NONE', #9794, #3613, #8268, .T. ) ;
#17283=CARTESIAN_POINT ( 'NONE',  ( 0.000000000000000000, -13.75000000000000533, 0.000000000000000000 ) ) ;
#17316=CARTESIAN_POINT ( 'NONE',  ( 10.04305231718605285, -26.50000000000000000, -33.55933677959240669 ) ) ;
#17331=VERTEX_POINT ( 'NONE', #15895 ) ;
#17332=FACE_OUTER_BOUND ( 'NONE', #6615, .T. ) ;
#17369=VERTEX_POINT ( 'NONE', #7122 ) ;
#17371=ORIENTED_EDGE ( 'NONE', *, *, #14953, .F. ) ;
#17409=DIRECTION ( 'NONE',  ( -0.000000000000000000, 1.000000000000000000, -0.000000000000000000 ) ) ;
#17419=DIRECTION ( 'NONE',  ( 0.9995004958639132076, 0.000000000000000000, 0.03160314490350067673 ) ) ;
#17450=CARTESIAN_POINT ( 'NONE',  ( 0.000000000000000000, -13.75000000000000355, 0.000000000000000000 ) ) ;
#17472=CYLINDRICAL_SURFACE ( 'NONE', #12473, 27.50000000000000000 ) ;
#17473=ORIENTED_EDGE ( 'NONE', *, *, #14448, .T. ) ;
#17474=ORIENTED_EDGE ( 'NONE', *, *, #16358, .F. ) ;
#17511=ORIENTED_EDGE ( 'NONE', *, *, #4957, .T. ) ;
#17518=DIRECTION ( 'NONE',  ( 0.000000000000000000, 0.000000000000000000, -1.000000000000000000 ) ) ;
#17527=CARTESIAN_POINT ( 'NONE',  ( 10.04305231718605285, -26.50000000000000000, -28.25933677959240953 ) ) ;
#17530=VECTOR ( 'NONE', #2045, 1000.000000000000000 ) ;
#17546=ORIENTED_EDGE ( 'NONE', *, *, #4591, .F. ) ;
#17548=AXIS2_PLACEMENT_3D ( 'NONE', #12772, #1252, #6852 ) ;
#17550=EDGE_LOOP ( 'NONE', ( #11624, #14422, #13157, #3845 ) ) ;
#17572=ORIENTED_EDGE ( 'NONE', *, *, #7563, .T. ) ;
#17624=ADVANCED_FACE ( 'NONE', ( #13146 ), #7513, .T. ) ;
#17644=( LENGTH_UNIT ( ) NAMED_UNIT ( * ) SI_UNIT ( .MILLI., .METRE. ) );
#17671=CARTESIAN_POINT ( 'NONE',  ( 0.000000000000000000, 11.24999999999999467, 0.000000000000000000 ) ) ;
#17673=ADVANCED_FACE ( 'NONE', ( #7610, #16553, #9505, #3422, #13427, #9216, #9414 ), #15319, .F. ) ;
#17738=DIRECTION ( 'NONE',  ( 0.000000000000000000, 1.000000000000000000, 0.000000000000000000 ) ) ;
#17785=CARTESIAN_POINT ( 'NONE',  ( 0.000000000000000000, 15.00000000000000000, 0.000000000000000000 ) ) ;
#17790=CARTESIAN_POINT ( 'NONE',  ( 10.04305231718605285, -26.50000000000000000, -28.25933677959240597 ) ) ;
#17808=AXIS2_PLACEMENT_3D ( 'NONE', #17450, #5914, #5830 ) ;
#17809=CARTESIAN_POINT ( 'NONE',  ( -0.3789929286210603765, 13.24999999999999822, 24.99712712213256438 ) ) ;
#17814=CARTESIAN_POINT ( 'NONE',  ( 10.04305231718605285, -30.00000000000000000, -33.55933677959240669 ) ) ;
#17816=CARTESIAN_POINT ( 'NONE',  ( -26.29305231718584324, -26.50000000000000000, 19.10302069950530779 ) ) ;
#17874=AXIS2_PLACEMENT_3D ( 'NONE', #3022, #18725, #2737 ) ;
#17892=ORIENTED_EDGE ( 'NONE', *, *, #7543, .F. ) ;
#17922=VECTOR ( 'NONE', #11999, 1000.000000000000000 ) ;
#17984=DIRECTION ( 'NONE',  ( 0.000000000000000000, 0.000000000000000000, 1.000000000000000000 ) ) ;
#18004=CARTESIAN_POINT ( 'NONE',  ( -26.29305231718568336, -26.50000000000000000, -21.75302069950551953 ) ) ;
#18060=EDGE_CURVE ( 'NONE', #9749, #16034, #1009, .T. ) ;
#18061=CARTESIAN_POINT ( 'NONE',  ( 0.000000000000000000, -17.25000000000000355, 27.50000000000000000 ) ) ;
#18069=DIRECTION ( 'NONE',  ( 0.000000000000000000, 1.000000000000000000, 0.000000000000000000 ) ) ;
#18074=DIRECTION ( 'NONE',  ( 0.000000000000000000, 0.000000000000000000, 1.000000000000000000 ) ) ;
#18105=VERTEX_POINT ( 'NONE', #6527 ) ;
#18110=CARTESIAN_POINT ( 'NONE',  ( -0.3789929286210603765, -30.00000000000000000, 24.99712712213256793 ) ) ;
#18139=VECTOR ( 'NONE', #5926, 1000.000000000000000 ) ;
#18153=FACE_OUTER_BOUND ( 'NONE', #576, .T. ) ;
#18171=EDGE_LOOP ( 'NONE', ( #9598, #10961, #15998, #8311 ) ) ;
#18203=CARTESIAN_POINT ( 'NONE',  ( 10.04305231718579705, -26.50000000000000000, 33.55933677959249195 ) ) ;
#18214=DIRECTION ( 'NONE',  ( 1.000000000000000000, 0.000000000000000000, 0.000000000000000000 ) ) ;
#18219=PLANE ( 'NONE',  #15448 ) ;
#18226=EDGE_CURVE ( 'NONE', #18412, #17183, #3138, .T. ) ;
#18272=ORIENTED_EDGE ( 'NONE', *, *, #18411, .T. ) ;
#18281=EDGE_LOOP ( 'NONE', ( #16402, #4918, #10811, #5581 ) ) ;
#18328=DIRECTION ( 'NONE',  ( -0.000000000000000000, 1.000000000000000000, -0.000000000000000000 ) ) ;
#18340=CYLINDRICAL_SURFACE ( 'NONE', #13999, 25.00000000000000000 ) ;
#18378=CARTESIAN_POINT ( 'NONE',  ( 3.367778697655221307E-15, -17.25000000000000355, -27.50000000000000000 ) ) ;
#18397=CARTESIAN_POINT ( 'NONE',  ( -26.29305231718584324, -26.50000000000000000, 21.75302069950530637 ) ) ;
#18411=EDGE_CURVE ( 'NONE', #5435, #5558, #10737, .T. ) ;
#18412=VERTEX_POINT ( 'NONE', #18623 ) ;
#18418=VECTOR ( 'NONE', #13411, 1000.000000000000000 ) ;
#18429=FACE_OUTER_BOUND ( 'NONE', #6627, .T. ) ;
#18449=AXIS2_PLACEMENT_3D ( 'NONE', #18476, #16671, #769 ) ;
#18451=DIRECTION ( 'NONE',  ( -0.000000000000000000, -1.000000000000000000, 0.000000000000000000 ) ) ;
#18452=DIRECTION ( 'NONE',  ( 0.000000000000000000, 0.000000000000000000, 1.000000000000000000 ) ) ;
#18457=ORIENTED_EDGE ( 'NONE', *, *, #7563, .F. ) ;
#18476=CARTESIAN_POINT ( 'NONE',  ( 0.000000000000000000, -30.00000000000000000, 0.000000000000000000 ) ) ;
#18499=CYLINDRICAL_SURFACE ( 'NONE', #13581, 41.00000000000000000 ) ;
#18506=DIRECTION ( 'NONE',  ( 1.000000000000000000, 0.000000000000000000, 0.000000000000000000 ) ) ;
#18514=AXIS2_PLACEMENT_3D ( 'NONE', #14990, #16141, #13279 ) ;
#18545=CARTESIAN_POINT ( 'NONE',  ( 0.000000000000000000, -30.00000000000000000, -41.00000000000000000 ) ) ;
#18623=CARTESIAN_POINT ( 'NONE',  ( -1.128893538851230005, 11.24999999999999467, 23.47286943213250154 ) ) ;
#18657=EDGE_CURVE ( 'NONE', #4975, #18105, #718, .T. ) ;
#18698=PRODUCT_CONTEXT ( 'NONE', #7187, 'mechanical' ) ;
#18725=DIRECTION ( 'NONE',  ( 0.000000000000000000, 1.000000000000000000, 0.000000000000000000 ) ) ;
#18727=EDGE_LOOP ( 'NONE', ( #8577, #3503, #15472, #3939 ) ) ;
#18744=DIRECTION ( 'NONE',  ( 0.000000000000000000, 1.000000000000000000, 0.000000000000000000 ) ) ;
#18776=AXIS2_PLACEMENT_3D ( 'NONE', #13880, #18451, #5411 ) ;
#18791=CIRCLE ( 'NONE', #17874, 27.50000000000000000 ) ;
#18805=EDGE_CURVE ( 'NONE', #10656, #10272, #15939, .T. ) ;
#18884=COLOUR_RGB('Off White',0.89,0.88,0.83);
#18885=FILL_AREA_STYLE_COLOUR('',#18884);
#18886=FILL_AREA_STYLE('',(#18885));
#18887=SURFACE_STYLE_FILL_AREA(#18886);
#18888=SURFACE_SIDE_STYLE('',(#18887));
#18889=SURFACE_STYLE_USAGE(.BOTH.,#18888);
#18890=PRESENTATION_STYLE_ASSIGNMENT((#18889));
ENDSEC;
END-ISO-10303-21;
